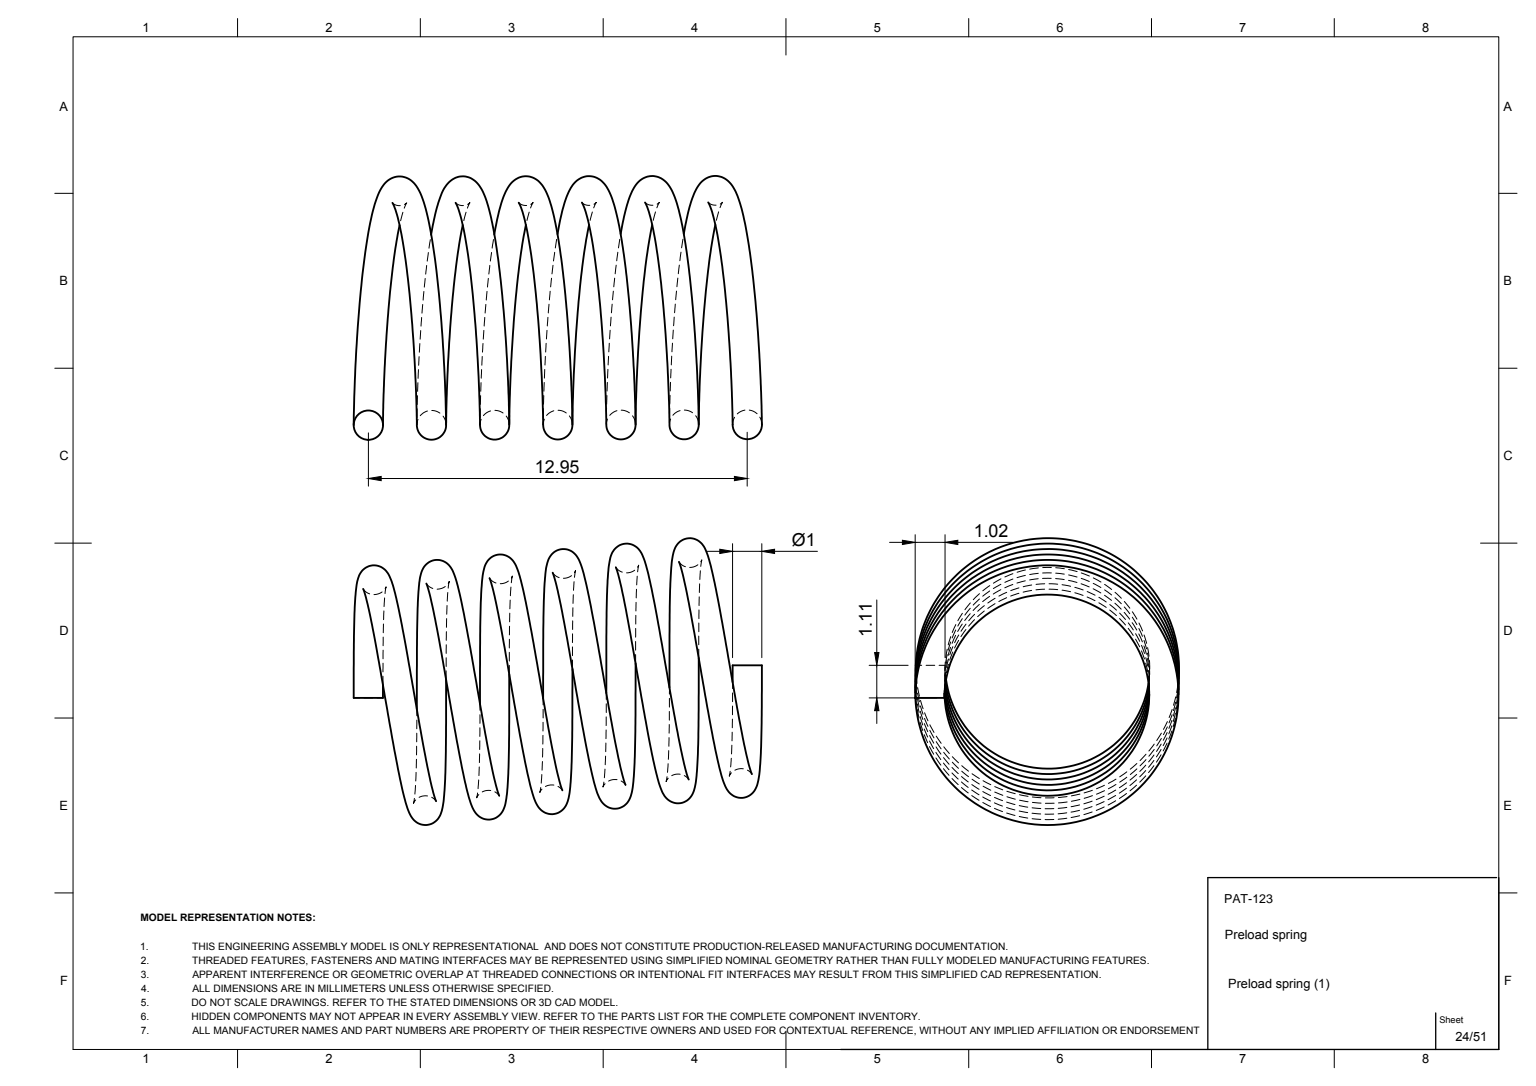
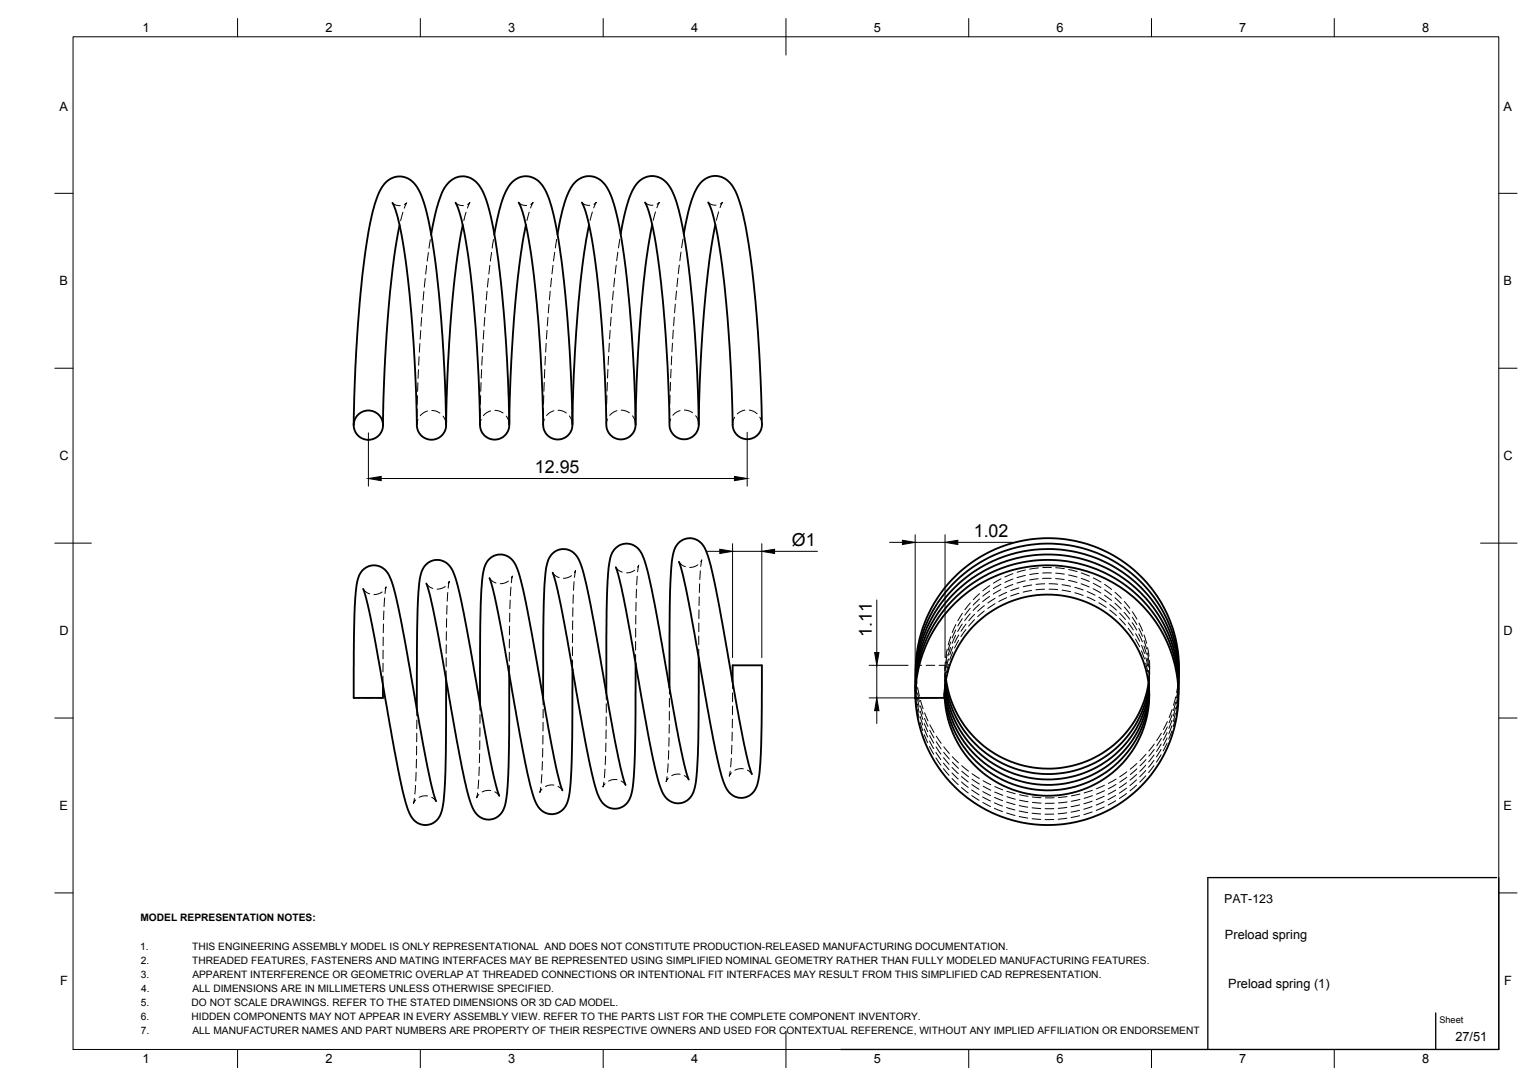
ISO-10303-21;
HEADER;
/* Generated by software containing ST-Developer
 * from STEP Tools, Inc. (www.steptools.com) 
 */

FILE_DESCRIPTION(
/* description */ ('Worm-less right-angle friction wheel drive'),
/* implementation_level */ '2;1');

FILE_NAME(
/* name */ 'Preload spring (1).step',
/* time_stamp */ '2026-10-28T03:22:36-07:00',
/* author */ (''),
/* organization */ (''),
/* preprocessor_version */ 'ST-DEVELOPER v20.2',
/* originating_system */ 'Autodesk Translation Framework v15.17.0.0',
/* authorisation */ '');

FILE_SCHEMA (('AUTOMOTIVE_DESIGN { 1 0 10303 214 3 1 1 }'));
ENDSEC;

DATA;
#10=MECHANICAL_DESIGN_GEOMETRIC_PRESENTATION_REPRESENTATION('',(#633),#17046);
#482=B_SPLINE_CURVE_WITH_KNOTS('',3,(#15240,#15241,#15242,#15243,#15244,
#15245,#15246,#15247,#15248,#15249,#15250,#15251,#15252,#15253,#15254,#15255,
#15256,#15257,#15258,#15259,#15260,#15261,#15262,#15263,#15264,#15265,#15266,
#15267,#15268,#15269,#15270,#15271,#15272,#15273,#15274,#15275,#15276,#15277,
#15278,#15279,#15280,#15281,#15282,#15283,#15284,#15285,#15286,#15287,#15288,
#15289,#15290,#15291,#15292,#15293,#15294,#15295,#15296,#15297,#15298,#15299,
#15300,#15301,#15302,#15303,#15304,#15305,#15306,#15307,#15308,#15309,#15310,
#15311,#15312,#15313,#15314,#15315,#15316,#15317,#15318,#15319,#15320),
 .UNSPECIFIED.,.F.,.F.,(4,1,1,1,1,1,1,1,1,1,1,1,1,1,1,1,1,1,1,1,1,1,1,1,
1,1,1,1,1,1,1,1,1,1,1,1,1,1,1,1,1,1,1,1,1,1,1,1,1,1,1,1,1,1,1,1,1,1,1,1,
1,1,1,1,1,1,1,1,1,1,1,1,1,1,1,1,1,1,4),(0.,0.00892857142857143,0.0178571428571429,
0.0357142857142857,0.0535714285714286,0.0714285714285714,0.0892857142857143,
0.107142857142857,0.125,0.142857142857143,0.158730158730159,0.174603174603175,
0.19047619047619,0.202380952380952,0.214285714285714,0.220238095238095,
0.226190476190476,0.238095238095238,0.25,0.261904761904762,0.273809523809524,
0.285714285714286,0.297619047619048,0.30952380952381,0.321428571428571,
0.333333333333333,0.349206349206349,0.365079365079365,0.376984126984127,
0.380952380952381,0.392857142857143,0.404761904761905,0.416666666666667,
0.428571428571429,0.446428571428571,0.464285714285714,0.476190476190476,
0.485119047619048,0.5,0.508928571428571,0.517857142857143,0.535714285714286,
0.553571428571429,0.571428571428571,0.589285714285714,0.607142857142857,
0.625,0.642857142857143,0.651785714285714,0.654761904761905,0.666666666666667,
0.678571428571428,0.696428571428571,0.705357142857143,0.714285714285714,
0.726190476190476,0.738095238095238,0.75,0.761904761904762,0.773809523809524,
0.785714285714286,0.797619047619047,0.803571428571428,0.806547619047619,
0.809523809523809,0.821428571428571,0.833333333333333,0.845238095238095,
0.857142857142857,0.866071428571429,0.875,0.892857142857143,0.910714285714286,
0.928571428571429,0.946428571428571,0.964285714285714,0.982142857142857,
0.991071428571429,1.),.UNSPECIFIED.);
#516=B_SPLINE_SURFACE_WITH_KNOTS('',3,3,((#14427,#14428,#14429,#14430,#14431,
#14432,#14433,#14434,#14435,#14436,#14437,#14438,#14439,#14440,#14441,#14442,
#14443,#14444,#14445,#14446,#14447,#14448,#14449,#14450,#14451,#14452,#14453,
#14454,#14455,#14456,#14457,#14458,#14459,#14460,#14461,#14462,#14463,#14464,
#14465,#14466,#14467,#14468,#14469,#14470,#14471,#14472,#14473,#14474,#14475,
#14476,#14477,#14478,#14479,#14480,#14481,#14482,#14483,#14484,#14485,#14486,
#14487,#14488,#14489,#14490,#14491,#14492,#14493,#14494,#14495,#14496,#14497,
#14498,#14499,#14500,#14501,#14502,#14503,#14504,#14505,#14506,#14507),
(#14508,#14509,#14510,#14511,#14512,#14513,#14514,#14515,#14516,#14517,
#14518,#14519,#14520,#14521,#14522,#14523,#14524,#14525,#14526,#14527,#14528,
#14529,#14530,#14531,#14532,#14533,#14534,#14535,#14536,#14537,#14538,#14539,
#14540,#14541,#14542,#14543,#14544,#14545,#14546,#14547,#14548,#14549,#14550,
#14551,#14552,#14553,#14554,#14555,#14556,#14557,#14558,#14559,#14560,#14561,
#14562,#14563,#14564,#14565,#14566,#14567,#14568,#14569,#14570,#14571,#14572,
#14573,#14574,#14575,#14576,#14577,#14578,#14579,#14580,#14581,#14582,#14583,
#14584,#14585,#14586,#14587,#14588),(#14589,#14590,#14591,#14592,#14593,
#14594,#14595,#14596,#14597,#14598,#14599,#14600,#14601,#14602,#14603,#14604,
#14605,#14606,#14607,#14608,#14609,#14610,#14611,#14612,#14613,#14614,#14615,
#14616,#14617,#14618,#14619,#14620,#14621,#14622,#14623,#14624,#14625,#14626,
#14627,#14628,#14629,#14630,#14631,#14632,#14633,#14634,#14635,#14636,#14637,
#14638,#14639,#14640,#14641,#14642,#14643,#14644,#14645,#14646,#14647,#14648,
#14649,#14650,#14651,#14652,#14653,#14654,#14655,#14656,#14657,#14658,#14659,
#14660,#14661,#14662,#14663,#14664,#14665,#14666,#14667,#14668,#14669),
(#14670,#14671,#14672,#14673,#14674,#14675,#14676,#14677,#14678,#14679,
#14680,#14681,#14682,#14683,#14684,#14685,#14686,#14687,#14688,#14689,#14690,
#14691,#14692,#14693,#14694,#14695,#14696,#14697,#14698,#14699,#14700,#14701,
#14702,#14703,#14704,#14705,#14706,#14707,#14708,#14709,#14710,#14711,#14712,
#14713,#14714,#14715,#14716,#14717,#14718,#14719,#14720,#14721,#14722,#14723,
#14724,#14725,#14726,#14727,#14728,#14729,#14730,#14731,#14732,#14733,#14734,
#14735,#14736,#14737,#14738,#14739,#14740,#14741,#14742,#14743,#14744,#14745,
#14746,#14747,#14748,#14749,#14750),(#14751,#14752,#14753,#14754,#14755,
#14756,#14757,#14758,#14759,#14760,#14761,#14762,#14763,#14764,#14765,#14766,
#14767,#14768,#14769,#14770,#14771,#14772,#14773,#14774,#14775,#14776,#14777,
#14778,#14779,#14780,#14781,#14782,#14783,#14784,#14785,#14786,#14787,#14788,
#14789,#14790,#14791,#14792,#14793,#14794,#14795,#14796,#14797,#14798,#14799,
#14800,#14801,#14802,#14803,#14804,#14805,#14806,#14807,#14808,#14809,#14810,
#14811,#14812,#14813,#14814,#14815,#14816,#14817,#14818,#14819,#14820,#14821,
#14822,#14823,#14824,#14825,#14826,#14827,#14828,#14829,#14830,#14831),
(#14832,#14833,#14834,#14835,#14836,#14837,#14838,#14839,#14840,#14841,
#14842,#14843,#14844,#14845,#14846,#14847,#14848,#14849,#14850,#14851,#14852,
#14853,#14854,#14855,#14856,#14857,#14858,#14859,#14860,#14861,#14862,#14863,
#14864,#14865,#14866,#14867,#14868,#14869,#14870,#14871,#14872,#14873,#14874,
#14875,#14876,#14877,#14878,#14879,#14880,#14881,#14882,#14883,#14884,#14885,
#14886,#14887,#14888,#14889,#14890,#14891,#14892,#14893,#14894,#14895,#14896,
#14897,#14898,#14899,#14900,#14901,#14902,#14903,#14904,#14905,#14906,#14907,
#14908,#14909,#14910,#14911,#14912),(#14913,#14914,#14915,#14916,#14917,
#14918,#14919,#14920,#14921,#14922,#14923,#14924,#14925,#14926,#14927,#14928,
#14929,#14930,#14931,#14932,#14933,#14934,#14935,#14936,#14937,#14938,#14939,
#14940,#14941,#14942,#14943,#14944,#14945,#14946,#14947,#14948,#14949,#14950,
#14951,#14952,#14953,#14954,#14955,#14956,#14957,#14958,#14959,#14960,#14961,
#14962,#14963,#14964,#14965,#14966,#14967,#14968,#14969,#14970,#14971,#14972,
#14973,#14974,#14975,#14976,#14977,#14978,#14979,#14980,#14981,#14982,#14983,
#14984,#14985,#14986,#14987,#14988,#14989,#14990,#14991,#14992,#14993),
(#14994,#14995,#14996,#14997,#14998,#14999,#15000,#15001,#15002,#15003,
#15004,#15005,#15006,#15007,#15008,#15009,#15010,#15011,#15012,#15013,#15014,
#15015,#15016,#15017,#15018,#15019,#15020,#15021,#15022,#15023,#15024,#15025,
#15026,#15027,#15028,#15029,#15030,#15031,#15032,#15033,#15034,#15035,#15036,
#15037,#15038,#15039,#15040,#15041,#15042,#15043,#15044,#15045,#15046,#15047,
#15048,#15049,#15050,#15051,#15052,#15053,#15054,#15055,#15056,#15057,#15058,
#15059,#15060,#15061,#15062,#15063,#15064,#15065,#15066,#15067,#15068,#15069,
#15070,#15071,#15072,#15073,#15074),(#15075,#15076,#15077,#15078,#15079,
#15080,#15081,#15082,#15083,#15084,#15085,#15086,#15087,#15088,#15089,#15090,
#15091,#15092,#15093,#15094,#15095,#15096,#15097,#15098,#15099,#15100,#15101,
#15102,#15103,#15104,#15105,#15106,#15107,#15108,#15109,#15110,#15111,#15112,
#15113,#15114,#15115,#15116,#15117,#15118,#15119,#15120,#15121,#15122,#15123,
#15124,#15125,#15126,#15127,#15128,#15129,#15130,#15131,#15132,#15133,#15134,
#15135,#15136,#15137,#15138,#15139,#15140,#15141,#15142,#15143,#15144,#15145,
#15146,#15147,#15148,#15149,#15150,#15151,#15152,#15153,#15154,#15155),
(#15156,#15157,#15158,#15159,#15160,#15161,#15162,#15163,#15164,#15165,
#15166,#15167,#15168,#15169,#15170,#15171,#15172,#15173,#15174,#15175,#15176,
#15177,#15178,#15179,#15180,#15181,#15182,#15183,#15184,#15185,#15186,#15187,
#15188,#15189,#15190,#15191,#15192,#15193,#15194,#15195,#15196,#15197,#15198,
#15199,#15200,#15201,#15202,#15203,#15204,#15205,#15206,#15207,#15208,#15209,
#15210,#15211,#15212,#15213,#15214,#15215,#15216,#15217,#15218,#15219,#15220,
#15221,#15222,#15223,#15224,#15225,#15226,#15227,#15228,#15229,#15230,#15231,
#15232,#15233,#15234,#15235,#15236)),.UNSPECIFIED.,.T.,.F.,.F.,(4,1,1,1,
1,1,1,4),(4,1,1,1,1,1,1,1,1,1,1,1,1,1,1,1,1,1,1,1,1,1,1,1,1,1,1,1,1,1,1,
1,1,1,1,1,1,1,1,1,1,1,1,1,1,1,1,1,1,1,1,1,1,1,1,1,1,1,1,1,1,1,1,1,1,1,1,
1,1,1,1,1,1,1,1,1,1,1,4),(-3.14159265358979,-2.24399475256414,-1.34639685153848,
-0.448798950512828,0.448798950512828,1.34639685153848,2.24399475256414,
3.14159265358979),(0.,0.00892857142857143,0.0178571428571429,0.0357142857142857,
0.0535714285714286,0.0714285714285714,0.0892857142857143,0.107142857142857,
0.125,0.142857142857143,0.158730158730159,0.174603174603175,0.19047619047619,
0.202380952380952,0.214285714285714,0.220238095238095,0.226190476190476,
0.238095238095238,0.25,0.261904761904762,0.273809523809524,0.285714285714286,
0.297619047619048,0.30952380952381,0.321428571428571,0.333333333333333,
0.349206349206349,0.365079365079365,0.376984126984127,0.380952380952381,
0.392857142857143,0.404761904761905,0.416666666666667,0.428571428571429,
0.446428571428571,0.464285714285714,0.476190476190476,0.485119047619048,
0.5,0.508928571428571,0.517857142857143,0.535714285714286,0.553571428571429,
0.571428571428571,0.589285714285714,0.607142857142857,0.625,0.642857142857143,
0.651785714285714,0.654761904761905,0.666666666666667,0.678571428571428,
0.696428571428571,0.705357142857143,0.714285714285714,0.726190476190476,
0.738095238095238,0.75,0.761904761904762,0.773809523809524,0.785714285714286,
0.797619047619047,0.803571428571428,0.806547619047619,0.809523809523809,
0.821428571428571,0.833333333333333,0.845238095238095,0.857142857142857,
0.866071428571429,0.875,0.892857142857143,0.910714285714286,0.928571428571429,
0.946428571428571,0.964285714285714,0.982142857142857,0.991071428571429,
1.),.UNSPECIFIED.);
#539=SHAPE_REPRESENTATION_RELATIONSHIP('SRR','None',#17282,#586);
#586=ADVANCED_BREP_SHAPE_REPRESENTATION('',(#687),#17018);
#633=STYLED_ITEM('',(#17591),#687);
#687=MANIFOLD_SOLID_BREP('Body1',#8188);
#1066=PLANE('',#9233);
#1067=PLANE('',#9234);
#1439=FACE_OUTER_BOUND('',#2095,.T.);
#1440=FACE_OUTER_BOUND('',#2096,.T.);
#1441=FACE_OUTER_BOUND('',#2097,.T.);
#2095=EDGE_LOOP('',(#6596,#6597,#6598,#6599));
#2096=EDGE_LOOP('',(#6600));
#2097=EDGE_LOOP('',(#6601));
#3691=CIRCLE('',#9231,0.05);
#3692=CIRCLE('',#9232,0.05);
#4223=VERTEX_POINT('',#15237);
#4224=VERTEX_POINT('',#15239);
#5067=EDGE_CURVE('',#4223,#4223,#3691,.T.);
#5068=EDGE_CURVE('',#4223,#4224,#482,.T.);
#5069=EDGE_CURVE('',#4224,#4224,#3692,.T.);
#6596=ORIENTED_EDGE('',*,*,#5067,.T.);
#6597=ORIENTED_EDGE('',*,*,#5068,.T.);
#6598=ORIENTED_EDGE('',*,*,#5069,.F.);
#6599=ORIENTED_EDGE('',*,*,#5068,.F.);
#6600=ORIENTED_EDGE('',*,*,#5069,.T.);
#6601=ORIENTED_EDGE('',*,*,#5067,.F.);
#7931=ADVANCED_FACE('',(#1439),#516,.T.);
#7932=ADVANCED_FACE('',(#1440),#1066,.T.);
#7933=ADVANCED_FACE('',(#1441),#1067,.F.);
#8188=CLOSED_SHELL('',(#7931,#7932,#7933));
#9230=AXIS2_PLACEMENT_3D('',#14426,#11045,#11046);
#9231=AXIS2_PLACEMENT_3D('',#15238,#11047,#11048);
#9232=AXIS2_PLACEMENT_3D('',#15321,#11049,#11050);
#9233=AXIS2_PLACEMENT_3D('',#15322,#11051,#11052);
#9234=AXIS2_PLACEMENT_3D('',#15323,#11053,#11054);
#11045=DIRECTION('axis',(0.,0.,1.));
#11046=DIRECTION('refdir',(1.,0.,0.));
#11047=DIRECTION('center_axis',(-0.000134420183300025,-0.085636011539688,
0.996326480356107));
#11048=DIRECTION('ref_axis',(1.1553650826854E-5,-0.996326489423811,-0.0856360107603029));
#11049=DIRECTION('center_axis',(0.000134419999317792,-0.085636011399563,
0.996326480368176));
#11050=DIRECTION('ref_axis',(0.0962365814952688,0.991703136101715,0.0852256430197378));
#11051=DIRECTION('center_axis',(0.000134419999317792,-0.085636011399563,
0.996326480368176));
#11052=DIRECTION('ref_axis',(0.0962365814952688,0.991703136101715,0.0852256430197378));
#11053=DIRECTION('center_axis',(-0.000134420183300025,-0.085636011539688,
0.996326480356107));
#11054=DIRECTION('ref_axis',(1.1553650826854E-5,-0.996326489423811,-0.0856360107603029));
#14426=CARTESIAN_POINT('',(0.,0.,0.));
#14427=CARTESIAN_POINT('Ctrl Pts',(5.89999942231746,7.09981632447119,4.00428180053801));
#14428=CARTESIAN_POINT('Ctrl Pts',(5.89999334367971,7.09594376396835,4.04933684813297));
#14429=CARTESIAN_POINT('Ctrl Pts',(5.88465017335476,7.08819405075721,4.13908165517953));
#14430=CARTESIAN_POINT('Ctrl Pts',(5.7964860030169,7.07263331806119,4.29968204261715));
#14431=CARTESIAN_POINT('Ctrl Pts',(5.59351456200701,7.05308119240215,4.4275031391656));
#14432=CARTESIAN_POINT('Ctrl Pts',(5.30510775645105,7.02945158726801,4.39546636939848));
#14433=CARTESIAN_POINT('Ctrl Pts',(5.09844717527872,7.00565845259414,4.18908156433879));
#14434=CARTESIAN_POINT('Ctrl Pts',(5.06491507736497,6.98170283632427,3.89688445847127));
#14435=CARTESIAN_POINT('Ctrl Pts',(5.22229231109316,6.957587725778,3.64598811283775));
#14436=CARTESIAN_POINT('Ctrl Pts',(5.50350105188817,6.93331581944121,3.54720017800962));
#14437=CARTESIAN_POINT('Ctrl Pts',(5.77606730494162,6.90979543600253,3.64243302852389));
#14438=CARTESIAN_POINT('Ctrl Pts',(5.93155863446605,6.88704927881041,3.87048202703801));
#14439=CARTESIAN_POINT('Ctrl Pts',(5.93201459027321,6.86509833940111,4.13672884061229));
#14440=CARTESIAN_POINT('Ctrl Pts',(5.79395734371705,6.84487476341531,4.33956419787309));
#14441=CARTESIAN_POINT('Ctrl Pts',(5.59585169142646,6.82641140225049,4.43472796239094));
#14442=CARTESIAN_POINT('Ctrl Pts',(5.43062330290708,6.81251496798271,4.43483227755276));
#14443=CARTESIAN_POINT('Ctrl Pts',(5.30781628774365,6.8013693608627,4.39175312056372));
#14444=CARTESIAN_POINT('Ctrl Pts',(5.19743069189207,6.79020509173472,4.32251414855249));
#14445=CARTESIAN_POINT('Ctrl Pts',(5.09353798605695,6.77621535562195,4.1924772803632));
#14446=CARTESIAN_POINT('Ctrl Pts',(5.04898925851302,6.75937456735607,3.99715324700454));
#14447=CARTESIAN_POINT('Ctrl Pts',(5.0935413464267,6.74248271039737,3.80123524176677));
#14448=CARTESIAN_POINT('Ctrl Pts',(5.21917592334569,6.72554188446977,3.64363320271165));
#14449=CARTESIAN_POINT('Ctrl Pts',(5.40122000385758,6.70855426693318,3.55590244763416));
#14450=CARTESIAN_POINT('Ctrl Pts',(5.60380955719718,6.6915221019177,3.55584448787041));
#14451=CARTESIAN_POINT('Ctrl Pts',(5.78691645390742,6.67444770371231,3.64394104146688));
#14452=CARTESIAN_POINT('Ctrl Pts',(5.91372041331327,6.65733344366189,3.80307026683985));
#14453=CARTESIAN_POINT('Ctrl Pts',(5.96466327221314,6.63827601600008,4.02414934139344));
#14454=CARTESIAN_POINT('Ctrl Pts',(5.88961383686182,6.61726302422527,4.26770951451258));
#14455=CARTESIAN_POINT('Ctrl Pts',(5.68975602864846,6.59619863118807,4.42707389952551));
#14456=CARTESIAN_POINT('Ctrl Pts',(5.50916223586277,6.58084997697241,4.45396467698472));
#14457=CARTESIAN_POINT('Ctrl Pts',(5.35453310810722,6.56740673736238,4.43070717074375));
#14458=CARTESIAN_POINT('Ctrl Pts',(5.21033393748589,6.55395079494006,4.36132595428699));
#14459=CARTESIAN_POINT('Ctrl Pts',(5.08177516019845,6.53662851034176,4.20021226638331));
#14460=CARTESIAN_POINT('Ctrl Pts',(5.03609211123456,6.51928717867399,3.99913913108666));
#14461=CARTESIAN_POINT('Ctrl Pts',(5.08928582945947,6.49903664031616,3.76419897777231));
#14462=CARTESIAN_POINT('Ctrl Pts',(5.28978283301087,6.47587070029814,3.56256415950519));
#14463=CARTESIAN_POINT('Ctrl Pts',(5.57279015344961,6.4526862562021,3.53101713469425));
#14464=CARTESIAN_POINT('Ctrl Pts',(5.7744501239661,6.4338421384389,3.62890875798563));
#14465=CARTESIAN_POINT('Ctrl Pts',(5.91107614262552,6.41644569471267,3.78134048060785));
#14466=CARTESIAN_POINT('Ctrl Pts',(5.96451577569518,6.40049895608791,3.96616344909838));
#14467=CARTESIAN_POINT('Ctrl Pts',(5.9327299609379,6.3845554854669,4.15104965949736));
#14468=CARTESIAN_POINT('Ctrl Pts',(5.83415684595966,6.36716688464879,4.33040203531341));
#14469=CARTESIAN_POINT('Ctrl Pts',(5.60855787080152,6.3454421500065,4.47243154476512));
#14470=CARTESIAN_POINT('Ctrl Pts',(5.29067075546292,6.31939963984916,4.43654609473001));
#14471=CARTESIAN_POINT('Ctrl Pts',(5.06495666340114,6.29339375333233,4.21070709279472));
#14472=CARTESIAN_POINT('Ctrl Pts',(5.02940089438198,6.26743382198568,3.89407398616837));
#14473=CARTESIAN_POINT('Ctrl Pts',(5.19880065125732,6.24152902171826,3.62471661866899));
#14474=CARTESIAN_POINT('Ctrl Pts',(5.49820781434257,6.21568834443117,3.52014376389726));
#14475=CARTESIAN_POINT('Ctrl Pts',(5.74701061020189,6.19421520170402,3.60728770872527));
#14476=CARTESIAN_POINT('Ctrl Pts',(5.85863359577984,6.17993370216935,3.73296424281348));
#14477=CARTESIAN_POINT('Ctrl Pts',(5.92288006435656,6.16852118154694,3.84896516413552));
#14478=CARTESIAN_POINT('Ctrl Pts',(5.95664235896203,6.15570021350747,3.99755228818456));
#14479=CARTESIAN_POINT('Ctrl Pts',(5.90422907170185,6.13580438066566,4.22863954557107));
#14480=CARTESIAN_POINT('Ctrl Pts',(5.74463079333177,6.1173884553624,4.38823789360272));
#14481=CARTESIAN_POINT('Ctrl Pts',(5.55259803695828,6.10044178794059,4.44287010078724));
#14482=CARTESIAN_POINT('Ctrl Pts',(5.38717753744307,6.08634982964905,4.43381260797737));
#14483=CARTESIAN_POINT('Ctrl Pts',(5.22149962135128,6.07088880373497,4.35387124517548));
#14484=CARTESIAN_POINT('Ctrl Pts',(5.09676922730111,6.0540743240685,4.197519449458));
#14485=CARTESIAN_POINT('Ctrl Pts',(5.0525318165955,6.03731392845979,4.00312051246728));
#14486=CARTESIAN_POINT('Ctrl Pts',(5.09677460214568,6.02060952469266,3.80936725739853));
#14487=CARTESIAN_POINT('Ctrl Pts',(5.22036100773764,6.00396293698029,3.65469518694587));
#14488=CARTESIAN_POINT('Ctrl Pts',(5.39815221757406,5.98737590584214,3.56901265908242));
#14489=CARTESIAN_POINT('Ctrl Pts',(5.56194673621828,5.9736043825902,3.56918712785721));
#14490=CARTESIAN_POINT('Ctrl Pts',(5.6678409475086,5.96399177625527,3.60634259138081));
#14491=CARTESIAN_POINT('Ctrl Pts',(5.72360710674561,5.9585067948969,3.63716464071472));
#14492=CARTESIAN_POINT('Ctrl Pts',(5.80152037634414,5.9502873075744,3.69239994875946));
#14493=CARTESIAN_POINT('Ctrl Pts',(5.89262775771971,5.93798818799799,3.80682412790902));
#14494=CARTESIAN_POINT('Ctrl Pts',(5.93588165070209,5.9216549676263,3.9962737943898));
#14495=CARTESIAN_POINT('Ctrl Pts',(5.89265315890838,5.90538862230925,4.18485446150754));
#14496=CARTESIAN_POINT('Ctrl Pts',(5.78249899819111,5.89054018760752,4.32296861862104));
#14497=CARTESIAN_POINT('Ctrl Pts',(5.64397324912796,5.87709200642215,4.39928196165792));
#14498=CARTESIAN_POINT('Ctrl Pts',(5.45729571883929,5.86100659113963,4.43140768516966));
#14499=CARTESIAN_POINT('Ctrl Pts',(5.22574876053333,5.84099901355926,4.35024097908663));
#14500=CARTESIAN_POINT('Ctrl Pts',(5.0699063365284,5.81715142001874,4.10208650989737));
#14501=CARTESIAN_POINT('Ctrl Pts',(5.10298913581097,5.79346725679344,3.81314318112568));
#14502=CARTESIAN_POINT('Ctrl Pts',(5.30729513304354,5.76994860790156,3.60917536341897));
#14503=CARTESIAN_POINT('Ctrl Pts',(5.59246492988907,5.74659517888843,3.57738640664907));
#14504=CARTESIAN_POINT('Ctrl Pts',(5.79284572265032,5.72727468967069,3.7038989587173));
#14505=CARTESIAN_POINT('Ctrl Pts',(5.8800308145667,5.71189869700794,3.86253471396896));
#14506=CARTESIAN_POINT('Ctrl Pts',(5.8951821641861,5.70424160396714,3.95121652410008));
#14507=CARTESIAN_POINT('Ctrl Pts',(5.89518817092524,5.70041484319491,3.99573871784903));
#14508=CARTESIAN_POINT('Ctrl Pts',(5.88503945743652,7.09981632447119,4.0042797822024));
#14509=CARTESIAN_POINT('Ctrl Pts',(5.88503360188162,7.09608588493208,4.04768133289771));
#14510=CARTESIAN_POINT('Ctrl Pts',(5.87026126699026,7.08862396394419,4.13409876124989));
#14511=CARTESIAN_POINT('Ctrl Pts',(5.78535030584819,7.07363703375696,4.28878882173021));
#14512=CARTESIAN_POINT('Ctrl Pts',(5.58981457160439,7.05480252942765,4.41195005833011));
#14513=CARTESIAN_POINT('Ctrl Pts',(5.31179486198712,7.03202561227573,4.38109726858311));
#14514=CARTESIAN_POINT('Ctrl Pts',(5.1124277587765,7.00907674704486,4.18203908678982));
#14515=CARTESIAN_POINT('Ctrl Pts',(5.08001803350251,6.98595417860409,3.8999761925135));
#14516=CARTESIAN_POINT('Ctrl Pts',(5.23203136694347,6.96266049576345,3.65754564919961));
#14517=CARTESIAN_POINT('Ctrl Pts',(5.50396936937568,6.93919148734548,3.56195831409131));
#14518=CARTESIAN_POINT('Ctrl Pts',(5.76786360761367,6.91642620730754,3.65410210166395));
#14519=CARTESIAN_POINT('Ctrl Pts',(5.91859875131219,6.89438580758112,3.87509306663505));
#14520=CARTESIAN_POINT('Ctrl Pts',(5.91908754056048,6.8730906966479,4.13341261767347));
#14521=CARTESIAN_POINT('Ctrl Pts',(5.78502683264549,6.85345041326714,4.33045812820945));
#14522=CARTESIAN_POINT('Ctrl Pts',(5.59240862903414,6.83550085128541,4.42301346486046));
#14523=CARTESIAN_POINT('Ctrl Pts',(5.43159993473068,6.82197903313836,4.42313220394627));
#14524=CARTESIAN_POINT('Ctrl Pts',(5.31198346558657,6.81112423395334,4.38117622245278));
#14525=CARTESIAN_POINT('Ctrl Pts',(5.20441120090185,6.80024507289894,4.31370604089673));
#14526=CARTESIAN_POINT('Ctrl Pts',(5.10308448889811,6.78660773456135,4.18691472624338));
#14527=CARTESIAN_POINT('Ctrl Pts',(5.05957333477074,6.7701692409416,3.99624133185818));
#14528=CARTESIAN_POINT('Ctrl Pts',(5.10308658178506,6.75366451037247,3.80477816416283));
#14529=CARTESIAN_POINT('Ctrl Pts',(5.22596911064028,6.73709691740872,3.65058727641187));
#14530=CARTESIAN_POINT('Ctrl Pts',(5.40424154502889,6.72046420161793,3.56464409931812));
#14531=CARTESIAN_POINT('Ctrl Pts',(5.60286757635272,6.70376966024345,3.56456110898369));
#14532=CARTESIAN_POINT('Ctrl Pts',(5.78260975317895,6.68701499206993,3.65100600925544));
#14533=CARTESIAN_POINT('Ctrl Pts',(5.90723898021823,6.67020103323329,3.80736557672115));
#14534=CARTESIAN_POINT('Ctrl Pts',(5.95739144160597,6.65145878281361,4.02485643420641));
#14535=CARTESIAN_POINT('Ctrl Pts',(5.88350382080552,6.63075660525971,4.26484435626206));
#14536=CARTESIAN_POINT('Ctrl Pts',(5.68632699032047,6.60997572305765,4.42215495861284));
#14537=CARTESIAN_POINT('Ctrl Pts',(5.50786242867171,6.59481082042869,4.44875398416139));
#14538=CARTESIAN_POINT('Ctrl Pts',(5.35492443239398,6.58151601836513,4.42575382239937));
#14539=CARTESIAN_POINT('Ctrl Pts',(5.21218195064913,6.56819993097658,4.35709671903736));
#14540=CARTESIAN_POINT('Ctrl Pts',(5.08473882673911,6.55103208305566,4.19743115221831));
#14541=CARTESIAN_POINT('Ctrl Pts',(5.03937938103974,6.53382903633989,3.9979075972426));
#14542=CARTESIAN_POINT('Ctrl Pts',(5.09219616215328,6.51371045047149,3.76446604094244));
#14543=CARTESIAN_POINT('Ctrl Pts',(5.29164216583296,6.49066863108082,3.56375987550904));
#14544=CARTESIAN_POINT('Ctrl Pts',(5.57380855674231,6.46755668746403,3.53221661138612));
#14545=CARTESIAN_POINT('Ctrl Pts',(5.77520948735709,6.44874487708301,3.62994883143992));
#14546=CARTESIAN_POINT('Ctrl Pts',(5.9118194085888,6.4313515231649,3.78234207954662));
#14547=CARTESIAN_POINT('Ctrl Pts',(5.96535290798642,6.41539494756269,3.96733324055338));
#14548=CARTESIAN_POINT('Ctrl Pts',(5.93350724448179,6.39941600080786,4.15265573762338));
#14549=CARTESIAN_POINT('Ctrl Pts',(5.83462795102543,6.38197230496921,4.3326009207179));
#14550=CARTESIAN_POINT('Ctrl Pts',(5.60802480207367,6.36015239803693,4.47536066940383));
#14551=CARTESIAN_POINT('Ctrl Pts',(5.28804071704905,6.33394375008401,4.43934003157992));
#14552=CARTESIAN_POINT('Ctrl Pts',(5.0603505371736,6.30772509227727,4.2116637907064));
#14553=CARTESIAN_POINT('Ctrl Pts',(5.02433426469034,6.28150024364713,3.89177497027619));
#14554=CARTESIAN_POINT('Ctrl Pts',(5.19569399285247,6.25529612930055,3.61911293303289));
#14555=CARTESIAN_POINT('Ctrl Pts',(5.49925070212339,6.22909620166617,3.51299220778051));
#14556=CARTESIAN_POINT('Ctrl Pts',(5.75197475889608,6.20729451095337,3.60142940412264));
#14557=CARTESIAN_POINT('Ctrl Pts',(5.86550798533523,6.19277158813603,3.72923955502794));
#14558=CARTESIAN_POINT('Ctrl Pts',(5.93088617148282,6.18115900724412,3.8472804234726));
#14559=CARTESIAN_POINT('Ctrl Pts',(5.96528306606778,6.16810503068496,3.99858218016166));
#14560=CARTESIAN_POINT('Ctrl Pts',(5.91188622152517,6.14782425772989,4.23416182125941));
#14561=CARTESIAN_POINT('Ctrl Pts',(5.7490193624655,6.12903078679408,4.39711001697646));
#14562=CARTESIAN_POINT('Ctrl Pts',(5.55277074738954,6.11171437387845,4.45295636322444));
#14563=CARTESIAN_POINT('Ctrl Pts',(5.38358725567555,6.09730363521905,4.44370269520848));
#14564=CARTESIAN_POINT('Ctrl Pts',(5.21398497489651,6.08147921618268,4.3618860003188));
#14565=CARTESIAN_POINT('Ctrl Pts',(5.08616324600684,6.06425310299918,4.20169628716414));
#14566=CARTESIAN_POINT('Ctrl Pts',(5.04077402087937,6.04706393365499,4.00231532025332));
#14567=CARTESIAN_POINT('Ctrl Pts',(5.08617032093218,6.02991837734054,3.80341237994541));
#14568=CARTESIAN_POINT('Ctrl Pts',(5.21314140461402,6.01281654577742,3.64447952839659));
#14569=CARTESIAN_POINT('Ctrl Pts',(5.39596558147649,5.99576114159946,3.55635140588749));
#14570=CARTESIAN_POINT('Ctrl Pts',(5.56454843416681,5.98158811350942,3.55651828149823));
#14571=CARTESIAN_POINT('Ctrl Pts',(5.67360413989068,5.97168893571421,3.59478043709277));
#14572=CARTESIAN_POINT('Ctrl Pts',(5.73105166386915,5.96603869488852,3.62653169595776));
#14573=CARTESIAN_POINT('Ctrl Pts',(5.8113292722746,5.95756999758158,3.68344222347348));
#14574=CARTESIAN_POINT('Ctrl Pts',(5.90525200105339,5.94489303633764,3.80138469729133));
#14575=CARTESIAN_POINT('Ctrl Pts',(5.9498859624265,5.92804546902486,3.99680740667185));
#14576=CARTESIAN_POINT('Ctrl Pts',(5.90527406073601,5.91125567170158,4.19147367065731));
#14577=CARTESIAN_POINT('Ctrl Pts',(5.79150254559316,5.89591895994826,4.33414205895609));
#14578=CARTESIAN_POINT('Ctrl Pts',(5.64834101429215,5.88202102372911,4.4130140624278));
#14579=CARTESIAN_POINT('Ctrl Pts',(5.4553346472487,5.86539043683629,4.44623569719961));
#14580=CARTESIAN_POINT('Ctrl Pts',(5.21578000821573,5.84469228785158,4.36229253299229));
#14581=CARTESIAN_POINT('Ctrl Pts',(5.05441367332187,5.82000362720346,4.10540136247045));
#14582=CARTESIAN_POINT('Ctrl Pts',(5.08866429485251,5.79546931039049,3.80607791306765));
#14583=CARTESIAN_POINT('Ctrl Pts',(5.30040509492993,5.77109351117434,3.59466769610795));
#14584=CARTESIAN_POINT('Ctrl Pts',(5.59608563803559,5.74687955036343,3.56169371934204));
#14585=CARTESIAN_POINT('Ctrl Pts',(5.80392030130352,5.72684060107471,3.69290766840958));
#14586=CARTESIAN_POINT('Ctrl Pts',(5.89435424813677,5.71089217884313,3.85744883447212));
#14587=CARTESIAN_POINT('Ctrl Pts',(5.91007247017572,5.70294882509164,3.94944546934017));
#14588=CARTESIAN_POINT('Ctrl Pts',(5.91007869895502,5.69898060743533,3.99561343380099));
#14589=CARTESIAN_POINT('Ctrl Pts',(5.85520827475736,7.08553591511819,4.00304833122987));
#14590=CARTESIAN_POINT('Ctrl Pts',(5.85520286590809,7.08209006146883,4.04313888631962));
#14591=CARTESIAN_POINT('Ctrl Pts',(5.84156747486463,7.07520486942886,4.12287606165967));
#14592=CARTESIAN_POINT('Ctrl Pts',(5.76326212603904,7.06138551553941,4.26551030037515));
#14593=CARTESIAN_POINT('Ctrl Pts',(5.58313571416996,7.04403789214147,4.37890493291776));
#14594=CARTESIAN_POINT('Ctrl Pts',(5.32733643620847,7.02308074340475,4.35047304239883));
#14595=CARTESIAN_POINT('Ctrl Pts',(5.14406551156473,7.00198204308889,4.16743848880527));
#14596=CARTESIAN_POINT('Ctrl Pts',(5.11430140308165,6.98073307206542,3.90823568037324));
#14597=CARTESIAN_POINT('Ctrl Pts',(5.2539756967838,6.9593299476571,3.68549505746316));
#14598=CARTESIAN_POINT('Ctrl Pts',(5.50385557975491,6.93776292440614,3.59765170680461));
#14599=CARTESIAN_POINT('Ctrl Pts',(5.746454002493,6.91683348560458,3.68233751904534));
#14600=CARTESIAN_POINT('Ctrl Pts',(5.88513081194609,6.89655721527044,3.8856066901103));
#14601=CARTESIAN_POINT('Ctrl Pts',(5.88561108039455,6.87695122617721,4.12342024789602));
#14602=CARTESIAN_POINT('Ctrl Pts',(5.7620912805646,6.85884906967209,4.30503249532845));
#14603=CARTESIAN_POINT('Ctrl Pts',(5.58439221890232,6.84228705858853,4.39044285766885));
#14604=CARTESIAN_POINT('Ctrl Pts',(5.43587731018536,6.82979711795253,4.39056857002489));
#14605=CARTESIAN_POINT('Ctrl Pts',(5.32531224002107,6.81976316059046,4.35179163381183));
#14606=CARTESIAN_POINT('Ctrl Pts',(5.22582219123238,6.80970122556429,4.28939485292107));
#14607=CARTESIAN_POINT('Ctrl Pts',(5.13200246986364,6.79707273454254,4.17202717151191));
#14608=CARTESIAN_POINT('Ctrl Pts',(5.09164094749547,6.78183341704652,3.99528331468449));
#14609=CARTESIAN_POINT('Ctrl Pts',(5.13200751743207,6.7665098094977,3.81754003421871));
#14610=CARTESIAN_POINT('Ctrl Pts',(5.24623575349236,6.75110199174121,3.67415956298011));
#14611=CARTESIAN_POINT('Ctrl Pts',(5.41224144571201,6.73560920651841,3.59409517730086));
#14612=CARTESIAN_POINT('Ctrl Pts',(5.59753307127925,6.72003176914412,3.59398376812156));
#14613=CARTESIAN_POINT('Ctrl Pts',(5.76552583542977,6.7043697251995,3.67473816518997));
#14614=CARTESIAN_POINT('Ctrl Pts',(5.88224637668914,6.68862335676344,3.82111570717619));
#14615=CARTESIAN_POINT('Ctrl Pts',(5.92933877872348,6.67103426452799,4.02514024338844));
#14616=CARTESIAN_POINT('Ctrl Pts',(5.85995562430613,6.65156702212541,4.25083041727868));
#14617=CARTESIAN_POINT('Ctrl Pts',(5.67407637808894,6.63196546184507,4.39925506328189));
#14618=CARTESIAN_POINT('Ctrl Pts',(5.50535216060145,6.61762539342909,4.42444600623728));
#14619=CARTESIAN_POINT('Ctrl Pts',(5.3605465743758,6.60503616153032,4.40267199067841));
#14620=CARTESIAN_POINT('Ctrl Pts',(5.22516696857318,6.59240538591147,4.33759897336023));
#14621=CARTESIAN_POINT('Ctrl Pts',(5.10399727465634,6.57608706132853,4.18587447130434));
#14622=CARTESIAN_POINT('Ctrl Pts',(5.06072881807943,6.55969079980481,3.9957755594979));
#14623=CARTESIAN_POINT('Ctrl Pts',(5.11111408899349,6.54047310824596,3.77281018900098));
#14624=CARTESIAN_POINT('Ctrl Pts',(5.30208506774464,6.51838444294906,3.58039325945438));
#14625=CARTESIAN_POINT('Ctrl Pts',(5.57344463256731,6.49615180944088,3.54987434760595));
#14626=CARTESIAN_POINT('Ctrl Pts',(5.76781931146614,6.47799290930932,3.64412456683428));
#14627=CARTESIAN_POINT('Ctrl Pts',(5.89995287193516,6.46117266087352,3.79146891932382));
#14628=CARTESIAN_POINT('Ctrl Pts',(5.95194793315776,6.44569200784306,3.97083844037072));
#14629=CARTESIAN_POINT('Ctrl Pts',(5.92101524437169,6.43015394352054,4.15103610674214));
#14630=CARTESIAN_POINT('Ctrl Pts',(5.82471537837473,6.41315680171824,4.32636138876989));
#14631=CARTESIAN_POINT('Ctrl Pts',(5.60334919178702,6.39182442975737,4.46603253787654));
#14632=CARTESIAN_POINT('Ctrl Pts',(5.28930632440049,6.36609845573924,4.43091101628552));
#14633=CARTESIAN_POINT('Ctrl Pts',(5.06476647708227,6.34025240232702,4.20670542372654));
#14634=CARTESIAN_POINT('Ctrl Pts',(5.02889907069948,6.3142971139968,3.89017648193371));
#14635=CARTESIAN_POINT('Ctrl Pts',(5.19901272516604,6.28823592961183,3.61906735374071));
#14636=CARTESIAN_POINT('Ctrl Pts',(5.50187330256082,6.26208782732235,3.51294889123812));
#14637=CARTESIAN_POINT('Ctrl Pts',(5.75522864687994,6.24022603278353,3.60140445329964));
#14638=CARTESIAN_POINT('Ctrl Pts',(5.8694004766967,6.22562326388648,3.72988152914194));
#14639=CARTESIAN_POINT('Ctrl Pts',(5.93521917425819,6.21393138166647,3.84871410099053));
#14640=CARTESIAN_POINT('Ctrl Pts',(5.9699545000092,6.2007640404577,4.00129391329599));
#14641=CARTESIAN_POINT('Ctrl Pts',(5.91603232645555,6.18025175472434,4.23954868417462));
#14642=CARTESIAN_POINT('Ctrl Pts',(5.75085163785764,6.16117154945629,4.40502717202795));
#14643=CARTESIAN_POINT('Ctrl Pts',(5.55107490688255,6.1435399111569,4.46192298098248));
#14644=CARTESIAN_POINT('Ctrl Pts',(5.37850386197236,6.12883720723606,4.45250910417445));
#14645=CARTESIAN_POINT('Ctrl Pts',(5.20506062246286,6.11265360212113,4.36891210542381));
#14646=CARTESIAN_POINT('Ctrl Pts',(5.07397022510475,6.09498817543275,4.20471986456681));
#14647=CARTESIAN_POINT('Ctrl Pts',(5.02724887723126,6.07731784476976,3.99979245739442));
#14648=CARTESIAN_POINT('Ctrl Pts',(5.07398000181797,6.05964215966279,3.79478075744986));
#14649=CARTESIAN_POINT('Ctrl Pts',(5.20512899117882,6.04196680287455,3.63051306675947));
#14650=CARTESIAN_POINT('Ctrl Pts',(5.39449791013073,6.02429430077605,3.53916197577409));
#14651=CARTESIAN_POINT('Ctrl Pts',(5.56957457418985,6.00957349714106,3.53928300415917));
#14652=CARTESIAN_POINT('Ctrl Pts',(5.68304311953453,5.99927347455427,3.57908441449588));
#14653=CARTESIAN_POINT('Ctrl Pts',(5.74286750570382,5.99338929587818,3.61214779557074));
#14654=CARTESIAN_POINT('Ctrl Pts',(5.82651752458846,5.98456439340875,3.67144751047707));
#14655=CARTESIAN_POINT('Ctrl Pts',(5.92457367352351,5.97133175061034,3.79451182749295));
#14656=CARTESIAN_POINT('Ctrl Pts',(5.97131861714195,5.95370439896441,3.99893579046224));
#14657=CARTESIAN_POINT('Ctrl Pts',(5.92459901326296,5.9360961851512,4.20307083437987));
#14658=CARTESIAN_POINT('Ctrl Pts',(5.80507236487523,5.91997636067228,4.35303796134367));
#14659=CARTESIAN_POINT('Ctrl Pts',(5.65434040611686,5.90534114871628,4.43611034923164));
#14660=CARTESIAN_POINT('Ctrl Pts',(5.45079337565466,5.88779962963185,4.47118188652743));
#14661=CARTESIAN_POINT('Ctrl Pts',(5.19748767042105,5.86591465359703,4.38257023322066));
#14662=CARTESIAN_POINT('Ctrl Pts',(5.0262253355364,5.83973026581737,4.1102456118929));
#14663=CARTESIAN_POINT('Ctrl Pts',(5.06249311301707,5.81363157422294,3.79188150756157));
#14664=CARTESIAN_POINT('Ctrl Pts',(5.28820296732657,5.78763167671582,3.56632359857709));
#14665=CARTESIAN_POINT('Ctrl Pts',(5.60433171174338,5.76173879777121,3.53092676719688));
#14666=CARTESIAN_POINT('Ctrl Pts',(5.8271423468097,5.74025670777543,3.67148617104396));
#14667=CARTESIAN_POINT('Ctrl Pts',(5.92424341235541,5.72313628975845,3.84810607771893));
#14668=CARTESIAN_POINT('Ctrl Pts',(5.94114425819813,5.71459769800728,3.94698841008634));
#14669=CARTESIAN_POINT('Ctrl Pts',(5.94115094957305,5.7103347709078,3.99658515196739));
#14670=CARTESIAN_POINT('Ctrl Pts',(5.8442633579502,7.03733205433023,3.99890364805841));
#14671=CARTESIAN_POINT('Ctrl Pts',(5.8442581197547,7.033994920285,4.03772931214518));
#14672=CARTESIAN_POINT('Ctrl Pts',(5.83104037018746,7.02733254813469,4.11486923947922));
#14673=CARTESIAN_POINT('Ctrl Pts',(5.75552618055734,7.01401654539893,4.25226823033117));
#14674=CARTESIAN_POINT('Ctrl Pts',(5.58280384378936,6.99739080062923,4.36069793188289));
#14675=CARTESIAN_POINT('Ctrl Pts',(5.33962002405483,6.97746235757696,4.33335540787856));
#14676=CARTESIAN_POINT('Ctrl Pts',(5.16682890132043,6.95754317780304,4.16039369672885));
#14677=CARTESIAN_POINT('Ctrl Pts',(5.13920853014916,6.93762223295465,3.91740209304229));
#14678=CARTESIAN_POINT('Ctrl Pts',(5.26947333563793,6.91768645343595,3.71016409897338));
#14679=CARTESIAN_POINT('Ctrl Pts',(5.50072401296219,6.89772870913039,3.62914290710299));
#14680=CARTESIAN_POINT('Ctrl Pts',(5.72372388246367,6.87847647854881,3.70723339336683));
#14681=CARTESIAN_POINT('Ctrl Pts',(5.85042194476176,6.85992603432529,3.89324231795015));
#14682=CARTESIAN_POINT('Ctrl Pts',(5.85070963937428,6.84207613283086,4.10972981319966));
#14683=CARTESIAN_POINT('Ctrl Pts',(5.73865422141122,6.82566665538221,4.27425669236962));
#14684=CARTESIAN_POINT('Ctrl Pts',(5.57815357745207,6.810706867649,4.35133307049917));
#14685=CARTESIAN_POINT('Ctrl Pts',(5.44441328362009,6.79945730366432,4.35140747521201));
#14686=CARTESIAN_POINT('Ctrl Pts',(5.34505646175606,6.79043938302152,4.31655337572742));
#14687=CARTESIAN_POINT('Ctrl Pts',(5.25576788953666,6.78140860275172,4.26054606594844));
#14688=CARTESIAN_POINT('Ctrl Pts',(5.1717433274605,6.77009209107834,4.15537468511295));
#14689=CARTESIAN_POINT('Ctrl Pts',(5.13570651291062,6.75647039032151,3.99739589300255));
#14690=CARTESIAN_POINT('Ctrl Pts',(5.17174572160623,6.74280160059864,3.83886918353745));
#14691=CARTESIAN_POINT('Ctrl Pts',(5.27346273046517,6.72908234649353,3.71124281622253));
#14692=CARTESIAN_POINT('Ctrl Pts',(5.42101179131082,6.71531148066912,3.6401110882049));
#14693=CARTESIAN_POINT('Ctrl Pts',(5.58544422096062,6.70148584866942,3.64003580689892));
#14694=CARTESIAN_POINT('Ctrl Pts',(5.73432346049268,6.68760313547377,3.71162565604183));
#14695=CARTESIAN_POINT('Ctrl Pts',(5.83764552929192,6.67366116797505,3.84122520535718));
#14696=CARTESIAN_POINT('Ctrl Pts',(5.87928444298638,6.658100912098,4.02169607449061));
#14697=CARTESIAN_POINT('Ctrl Pts',(5.81794296845177,6.64089543827006,4.22115320816706));
#14698=CARTESIAN_POINT('Ctrl Pts',(5.6537487144978,6.62358017931584,4.35224741413031));
#14699=CARTESIAN_POINT('Ctrl Pts',(5.50474573233506,6.61091566681907,4.37449449482154));
#14700=CARTESIAN_POINT('Ctrl Pts',(5.3768646872216,6.59979765360415,4.35526579110611));
#14701=CARTESIAN_POINT('Ctrl Pts',(5.25729954874086,6.58864209789496,4.29779828729648));
#14702=CARTESIAN_POINT('Ctrl Pts',(5.15025342040901,6.5742265315835,4.16377038217943));
#14703=CARTESIAN_POINT('Ctrl Pts',(5.11200030526049,6.55973534828414,3.99576364180229));
#14704=CARTESIAN_POINT('Ctrl Pts',(5.15654185679476,6.54274034280373,3.79858438441201));
#14705=CARTESIAN_POINT('Ctrl Pts',(5.32554784904026,6.52318707054893,3.62821328392619));
#14706=CARTESIAN_POINT('Ctrl Pts',(5.56613353860405,6.50347523010832,3.60107938902761));
#14707=CARTESIAN_POINT('Ctrl Pts',(5.73877029295882,6.48734943548394,3.68475125508372));
#14708=CARTESIAN_POINT('Ctrl Pts',(5.85627571304628,6.47239252636156,3.81575918380156));
#14709=CARTESIAN_POINT('Ctrl Pts',(5.90263031720046,6.45860635937458,3.97548974074165));
#14710=CARTESIAN_POINT('Ctrl Pts',(5.87505167436944,6.44474372928567,4.13626778107872));
#14711=CARTESIAN_POINT('Ctrl Pts',(5.78903514141083,6.42955803390157,4.29291835106576));
#14712=CARTESIAN_POINT('Ctrl Pts',(5.59088448553645,6.41045798350198,4.41808744129809));
#14713=CARTESIAN_POINT('Ctrl Pts',(5.30873518287549,6.38734750124527,4.38670311299745));
#14714=CARTESIAN_POINT('Ctrl Pts',(5.10615471140587,6.36404684857898,4.18468451257222));
#14715=CARTESIAN_POINT('Ctrl Pts',(5.07349898841052,6.34055522359989,3.8982098092804));
#14716=CARTESIAN_POINT('Ctrl Pts',(5.22791505782553,6.31687679944705,3.65170107095422));
#14717=CARTESIAN_POINT('Ctrl Pts',(5.50431592493739,6.29300768975538,3.55461983394832));
#14718=CARTESIAN_POINT('Ctrl Pts',(5.73671787489177,6.27296418176745,3.6355503842994));
#14719=CARTESIAN_POINT('Ctrl Pts',(5.84183688606317,6.25952452604128,3.75378707156832));
#14720=CARTESIAN_POINT('Ctrl Pts',(5.90252063540586,6.24874582138889,3.86334104486593));
#14721=CARTESIAN_POINT('Ctrl Pts',(5.93466081634591,6.23658242737163,4.00429106496237));
#14722=CARTESIAN_POINT('Ctrl Pts',(5.88477257211492,6.21756897840495,4.22516592599398));
#14723=CARTESIAN_POINT('Ctrl Pts',(5.73112374226898,6.19980983242131,4.37935499119927));
#14724=CARTESIAN_POINT('Ctrl Pts',(5.54437866031431,6.18333055162171,4.43259622705531));
#14725=CARTESIAN_POINT('Ctrl Pts',(5.38261999067874,6.16955106486449,4.42380810286847));
#14726=CARTESIAN_POINT('Ctrl Pts',(5.21948440418905,6.15433461785036,4.34526151688322));
#14727=CARTESIAN_POINT('Ctrl Pts',(5.09567527200945,6.13766356859339,4.19033418142023));
#14728=CARTESIAN_POINT('Ctrl Pts',(5.05132292060661,6.120920804985,3.99616808757238));
#14729=CARTESIAN_POINT('Ctrl Pts',(5.09568013075446,6.10411152452373,3.80114024004156));
#14730=CARTESIAN_POINT('Ctrl Pts',(5.2208564304236,6.08723548924311,3.64421655461967));
#14731=CARTESIAN_POINT('Ctrl Pts',(5.40236843774688,6.07029554676657,3.55655082292256));
#14732=CARTESIAN_POINT('Ctrl Pts',(5.57090761649076,6.05612632794669,3.55659431162632));
#14733=CARTESIAN_POINT('Ctrl Pts',(5.68047831247714,6.04618144828711,3.59501288603736));
#14734=CARTESIAN_POINT('Ctrl Pts',(5.7383337836807,6.04049119521234,3.62698653839934));
#14735=CARTESIAN_POINT('Ctrl Pts',(5.8193132044321,6.03194870990487,3.68438770351889));
#14736=CARTESIAN_POINT('Ctrl Pts',(5.91452854847537,6.0191093147926,3.80377513400947));
#14737=CARTESIAN_POINT('Ctrl Pts',(5.96017726931528,6.00193511332281,4.00295549686061));
#14738=CARTESIAN_POINT('Ctrl Pts',(5.91454763656368,5.98470857921717,4.2027269727812));
#14739=CARTESIAN_POINT('Ctrl Pts',(5.79716877045588,5.96887147306035,4.35014107428084));
#14740=CARTESIAN_POINT('Ctrl Pts',(5.64852424861931,5.95443918265348,4.43210799719531));
#14741=CARTESIAN_POINT('Ctrl Pts',(5.44716731617039,5.93708678955292,4.46686180108763));
#14742=CARTESIAN_POINT('Ctrl Pts',(5.19528800450862,5.91533634052886,4.37903445531321));
#14743=CARTESIAN_POINT('Ctrl Pts',(5.02367424394978,5.88914912040216,4.10682213449717));
#14744=CARTESIAN_POINT('Ctrl Pts',(5.05983407646609,5.86288698339694,3.78630359033442));
#14745=CARTESIAN_POINT('Ctrl Pts',(5.28822019826199,5.83655644865667,3.55758071132317));
#14746=CARTESIAN_POINT('Ctrl Pts',(5.61042287602758,5.81016939852405,3.52114893229972));
#14747=CARTESIAN_POINT('Ctrl Pts',(5.83908979198061,5.78814211888601,3.66511277419047));
#14748=CARTESIAN_POINT('Ctrl Pts',(5.93920546082742,5.77050202961558,3.8470873725861));
#14749=CARTESIAN_POINT('Ctrl Pts',(5.95669478049843,5.76167432127745,3.94932370527045));
#14750=CARTESIAN_POINT('Ctrl Pts',(5.95670170074323,5.75726558623602,4.00061683995683));
#14751=CARTESIAN_POINT('Ctrl Pts',(5.87514548417672,6.99854044864851,3.99557360787966));
#14752=CARTESIAN_POINT('Ctrl Pts',(5.87513978765661,6.99491132651841,4.03779638791872));
#14753=CARTESIAN_POINT('Ctrl Pts',(5.86075022359954,6.98766329031147,4.12172125899622));
#14754=CARTESIAN_POINT('Ctrl Pts',(5.77883107645889,6.97322759641233,4.27068148293984));
#14755=CARTESIAN_POINT('Ctrl Pts',(5.59230633485985,6.95528685852212,4.38753321295925));
#14756=CARTESIAN_POINT('Ctrl Pts',(5.33155020564179,6.93391865832403,4.35791618403263));
#14757=CARTESIAN_POINT('Ctrl Pts',(5.14773246729608,6.91270540416619,4.17347705756876));
#14758=CARTESIAN_POINT('Ctrl Pts',(5.11883580759173,6.89164103056227,3.9164440087751));
#14759=CARTESIAN_POINT('Ctrl Pts',(5.25588116695966,6.87071957668565,3.6990566497247));
#14760=CARTESIAN_POINT('Ctrl Pts',(5.49694403853312,6.84993083868618,3.6149532499762));
#14761=CARTESIAN_POINT('Ctrl Pts',(5.72739217434572,6.83003349550605,3.69599197049964));
#14762=CARTESIAN_POINT('Ctrl Pts',(5.85719964701457,6.81100327064808,3.88700464630704));
#14763=CARTESIAN_POINT('Ctrl Pts',(5.85726081296606,6.79281909841024,4.10758802917809));
#14764=CARTESIAN_POINT('Ctrl Pts',(5.74373291807669,6.77622423972196,4.27389444303247));
#14765=CARTESIAN_POINT('Ctrl Pts',(5.58236852338651,6.76119137058875,4.35125834030399));
#14766=CARTESIAN_POINT('Ctrl Pts',(5.44867419960033,6.74994884661536,4.35125385557247));
#14767=CARTESIAN_POINT('Ctrl Pts',(5.34976030800238,6.74097144095651,4.31653614511533));
#14768=CARTESIAN_POINT('Ctrl Pts',(5.26110773818199,6.73200480430205,4.26090950185114));
#14769=CARTESIAN_POINT('Ctrl Pts',(5.17808610936031,6.72081958457785,4.15686365468362));
#14770=CARTESIAN_POINT('Ctrl Pts',(5.1427384642525,6.70742370332015,4.00146629817937));
#14771=CARTESIAN_POINT('Ctrl Pts',(5.17808628986628,6.69405440549435,3.84640454479009));
#14772=CARTESIAN_POINT('Ctrl Pts',(5.27713337356397,6.68070956969354,3.72228233330786));
#14773=CARTESIAN_POINT('Ctrl Pts',(5.41998780176605,6.66738391686113,3.6535162350639));
#14774=CARTESIAN_POINT('Ctrl Pts',(5.57831764719913,6.65407511732755,3.65353579167895));
#14775=CARTESIAN_POINT('Ctrl Pts',(5.72089719398017,6.64077986955346,3.72219848416115));
#14776=CARTESIAN_POINT('Ctrl Pts',(5.81930953143935,6.62749439614206,3.84577722805825));
#14777=CARTESIAN_POINT('Ctrl Pts',(5.85870394850306,6.61274185884821,4.01697267297566));
#14778=CARTESIAN_POINT('Ctrl Pts',(5.80067105304151,6.59651509694839,4.20503754829806));
#14779=CARTESIAN_POINT('Ctrl Pts',(5.64666780825017,6.58028993315573,4.32776333798744));
#14780=CARTESIAN_POINT('Ctrl Pts',(5.50774076906622,6.56848394985099,4.34843470371925));
#14781=CARTESIAN_POINT('Ctrl Pts',(5.38885142963878,6.55814860077465,4.33055181655375));
#14782=CARTESIAN_POINT('Ctrl Pts',(5.27804026744975,6.54780951370302,4.2772266172093));
#14783=CARTESIAN_POINT('Ctrl Pts',(5.17927293647025,6.53450161770272,4.15344678062057));
#14784=CARTESIAN_POINT('Ctrl Pts',(5.14416812305239,6.52118046944049,3.99895936753469));
#14785=CARTESIAN_POINT('Ctrl Pts',(5.1850453990095,6.50561478324366,3.81835726355173));
#14786=CARTESIAN_POINT('Ctrl Pts',(5.339284997864,6.48779307370435,3.66315400412196));
#14787=CARTESIAN_POINT('Ctrl Pts',(5.55754831918104,6.46991368775191,3.63872503876236));
#14788=CARTESIAN_POINT('Ctrl Pts',(5.71350848036609,6.45534555587482,3.71438173891507));
#14789=CARTESIAN_POINT('Ctrl Pts',(5.81940093081938,6.44186425747974,3.83248890666509));
#14790=CARTESIAN_POINT('Ctrl Pts',(5.86099636209716,6.42947631893566,3.97607363283317));
#14791=CARTESIAN_POINT('Ctrl Pts',(5.83624924861445,6.41704875670862,4.12020838390855));
#14792=CARTESIAN_POINT('Ctrl Pts',(5.75924576580022,6.40345957109736,4.26039065665031));
#14793=CARTESIAN_POINT('Ctrl Pts',(5.58230732141824,6.38641243046477,4.37202924255808));
#14794=CARTESIAN_POINT('Ctrl Pts',(5.33119627254454,6.36584482021927,4.34397642119019));
#14795=CARTESIAN_POINT('Ctrl Pts',(5.15140636995601,6.34515949086949,4.16454562210437));
#14796=CARTESIAN_POINT('Ctrl Pts',(5.12254982607975,6.32434519787953,3.91070033361363));
#14797=CARTESIAN_POINT('Ctrl Pts',(5.25920873518247,6.30340142939672,3.6926602572414));
#14798=CARTESIAN_POINT('Ctrl Pts',(5.50347393537872,6.28230883810381,3.60690759285009));
#14799=CARTESIAN_POINT('Ctrl Pts',(5.70869616727121,6.26461043075207,3.67839455761512));
#14800=CARTESIAN_POINT('Ctrl Pts',(5.80150749996396,6.2527445027482,3.78278841553677));
#14801=CARTESIAN_POINT('Ctrl Pts',(5.8550859977429,6.24322788838423,3.87951569410302));
#14802=CARTESIAN_POINT('Ctrl Pts',(5.88346434910103,6.23248866320778,4.00396460760673));
#14803=CARTESIAN_POINT('Ctrl Pts',(5.83941409539019,6.21569758858433,4.19902206859976));
#14804=CARTESIAN_POINT('Ctrl Pts',(5.70367326626789,6.20000650214883,4.33527098884019));
#14805=CARTESIAN_POINT('Ctrl Pts',(5.53855228655731,6.18543517970738,4.38235651612384));
#14806=CARTESIAN_POINT('Ctrl Pts',(5.39543801792977,6.17324367379672,4.37458667586454));
#14807=CARTESIAN_POINT('Ctrl Pts',(5.25098024432611,6.15976998349194,4.30505194274034));
#14808=CARTESIAN_POINT('Ctrl Pts',(5.14121655731439,6.14499160555445,4.16773264727778));
#14809=CARTESIAN_POINT('Ctrl Pts',(5.10182587914745,6.13013154458964,3.99540643427926));
#14810=CARTESIAN_POINT('Ctrl Pts',(5.14122514831917,6.11519028373789,3.8220564397272));
#14811=CARTESIAN_POINT('Ctrl Pts',(5.25263588248017,6.10016628060021,3.68233820392778));
#14812=CARTESIAN_POINT('Ctrl Pts',(5.41448657988468,6.08505886588137,3.60412985666001));
#14813=CARTESIAN_POINT('Ctrl Pts',(5.56506704731687,6.07239919129658,3.60413578617919));
#14814=CARTESIAN_POINT('Ctrl Pts',(5.66311283101293,6.06350038653797,3.63850704060478));
#14815=CARTESIAN_POINT('Ctrl Pts',(5.7149221186375,6.05840477958295,3.66713842572877));
#14816=CARTESIAN_POINT('Ctrl Pts',(5.78747702938897,6.05075080923013,3.7185669337241));
#14817=CARTESIAN_POINT('Ctrl Pts',(5.87293025946013,6.03923050065618,3.82566146039982));
#14818=CARTESIAN_POINT('Ctrl Pts',(5.91402507704787,6.02378513403553,4.00476477146208));
#14819=CARTESIAN_POINT('Ctrl Pts',(5.87294369145138,6.00825508165675,4.18486099195512));
#14820=CARTESIAN_POINT('Ctrl Pts',(5.76690353827561,5.99394133612039,4.31811566915106));
#14821=CARTESIAN_POINT('Ctrl Pts',(5.63226512122908,5.98086723592559,4.39238906025841));
#14822=CARTESIAN_POINT('Ctrl Pts',(5.44950474947794,5.96511502927026,4.42397005765718));
#14823=CARTESIAN_POINT('Ctrl Pts',(5.22008211053465,5.94530667428613,4.34415650242552));
#14824=CARTESIAN_POINT('Ctrl Pts',(5.06291182507567,5.92134913814384,4.09528547532897));
#14825=CARTESIAN_POINT('Ctrl Pts',(5.09590900327192,5.89720669469332,3.80066624542902));
#14826=CARTESIAN_POINT('Ctrl Pts',(5.30668586808294,5.87288210191658,3.58923668118618));
#14827=CARTESIAN_POINT('Ctrl Pts',(5.60579413240307,5.84838086936144,3.55513713761874));
#14828=CARTESIAN_POINT('Ctrl Pts',(5.81936747109835,5.82781552400804,3.68933059315267));
#14829=CARTESIAN_POINT('Ctrl Pts',(5.91324358998992,5.81128381242343,3.85984598368901));
#14830=CARTESIAN_POINT('Ctrl Pts',(5.92970378689351,5.80298590584205,3.95593351696052));
#14831=CARTESIAN_POINT('Ctrl Pts',(5.92971029794461,5.79883785906193,4.00419369140481));
#14832=CARTESIAN_POINT('Ctrl Pts',(5.92479734822298,6.99869271407564,3.99559339418157));
#14833=CARTESIAN_POINT('Ctrl Pts',(5.92479090997151,6.99459105192559,4.04331390965279));
#14834=CARTESIAN_POINT('Ctrl Pts',(5.90850975380561,6.98638756199577,4.1382994503635));
#14835=CARTESIAN_POINT('Ctrl Pts',(5.8157856671956,6.97004679073908,4.30691427794729));
#14836=CARTESIAN_POINT('Ctrl Pts',(5.60456312519679,6.94972761837475,4.43926282438681));
#14837=CARTESIAN_POINT('Ctrl Pts',(5.30924514470025,6.92552625657262,4.40571412404912));
#14838=CARTESIAN_POINT('Ctrl Pts',(5.10115155224644,6.90150776708021,4.19688142095042));
#14839=CARTESIAN_POINT('Ctrl Pts',(5.06851049643939,6.87767566403273,3.90609185048507));
#14840=CARTESIAN_POINT('Ctrl Pts',(5.22342892068834,6.85403159761471,3.66049532779896));
#14841=CARTESIAN_POINT('Ctrl Pts',(5.49540131761851,6.8305770702376,3.56571109549459));
#14842=CARTESIAN_POINT('Ctrl Pts',(5.75478373950727,6.80817442310058,3.65704418598113));
#14843=CARTESIAN_POINT('Ctrl Pts',(5.90047506910969,6.78680000659775,3.8716090579534));
#14844=CARTESIAN_POINT('Ctrl Pts',(5.90043765469484,6.76643101559881,4.11867588537419));
#14845=CARTESIAN_POINT('Ctrl Pts',(5.77356623131722,6.7478962216523,4.30433440185149));
#14846=CARTESIAN_POINT('Ctrl Pts',(5.59386479707093,6.73115456608272,4.39041942156343));
#14847=CARTESIAN_POINT('Ctrl Pts',(5.44539655895096,6.71866722776999,4.39036886564142));
#14848=CARTESIAN_POINT('Ctrl Pts',(5.33579942713953,6.70871882259051,4.35189016716179));
#14849=CARTESIAN_POINT('Ctrl Pts',(5.23771902383275,6.69879786668875,4.2903366305777));
#14850=CARTESIAN_POINT('Ctrl Pts',(5.14611136868914,6.686446054238,4.17544171847082));
#14851=CARTESIAN_POINT('Ctrl Pts',(5.10728479879167,6.67170559659797,4.00445121458595));
#14852=CARTESIAN_POINT('Ctrl Pts',(5.14611211950831,6.65704405744421,3.83444276345394));
#14853=CARTESIAN_POINT('Ctrl Pts',(5.25438505285132,6.64245966977581,3.69887894687364));
#14854=CARTESIAN_POINT('Ctrl Pts',(5.40990166233343,6.62795227611534,3.62410389391192));
#14855=CARTESIAN_POINT('Ctrl Pts',(5.5815496819327,6.61351997914256,3.62420401324371));
#14856=CARTESIAN_POINT('Ctrl Pts',(5.73544946394382,6.59916119992895,3.69841415911542));
#14857=CARTESIAN_POINT('Ctrl Pts',(5.84118479017196,6.58487472963496,3.83131690200048));
#14858=CARTESIAN_POINT('Ctrl Pts',(5.88325122365517,6.56907782799123,4.01459123943289));
#14859=CARTESIAN_POINT('Ctrl Pts',(5.82128683856772,6.55180183670017,4.21474716794292));
#14860=CARTESIAN_POINT('Ctrl Pts',(5.65822534686918,6.53463077872286,4.34442789266045));
#14861=CARTESIAN_POINT('Ctrl Pts',(5.51207474544734,6.52220844326274,4.36609029268673));
#14862=CARTESIAN_POINT('Ctrl Pts',(5.38742554303644,6.51137100417828,4.34733263783343));
#14863=CARTESIAN_POINT('Ctrl Pts',(5.27165764889733,6.50056364797766,4.2915430638631));
#14864=CARTESIAN_POINT('Ctrl Pts',(5.16905588565897,6.48672787446753,4.16279863377245));
#14865=CARTESIAN_POINT('Ctrl Pts',(5.13283917983621,6.47294482309939,4.00299700475136));
#14866=CARTESIAN_POINT('Ctrl Pts',(5.1750114352257,6.45692788066795,3.81720051065741));
#14867=CARTESIAN_POINT('Ctrl Pts',(5.33289108133986,6.43870149704958,3.65876416560081));
#14868=CARTESIAN_POINT('Ctrl Pts',(5.55419693287486,6.42057082795549,3.63430277213249));
#14869=CARTESIAN_POINT('Ctrl Pts',(5.71118304201485,6.40589452371311,3.71057513225082));
#14870=CARTESIAN_POINT('Ctrl Pts',(5.81726355608341,6.39238507064568,3.82897080987877));
#14871=CARTESIAN_POINT('Ctrl Pts',(5.85858981339439,6.38003097260466,3.97213930596044));
#14872=CARTESIAN_POINT('Ctrl Pts',(5.83401059568513,6.36771004387122,4.11499949089278));
#14873=CARTESIAN_POINT('Ctrl Pts',(5.75793177724685,6.35429201109606,4.25337987346692));
#14874=CARTESIAN_POINT('Ctrl Pts',(5.5841434597572,6.33755678598937,4.36270673919398));
#14875=CARTESIAN_POINT('Ctrl Pts',(5.33972856653595,6.31752970311076,4.33506481527608));
#14876=CARTESIAN_POINT('Ctrl Pts',(5.16631525257735,6.29754423858894,4.16154035829682));
#14877=CARTESIAN_POINT('Ctrl Pts',(5.1389670014894,6.27759361927993,3.91823011012584));
#14878=CARTESIAN_POINT('Ctrl Pts',(5.26923427006138,6.25765586167643,3.71098251993868));
#14879=CARTESIAN_POINT('Ctrl Pts',(5.49997414943137,6.2377376533677,3.63028623162157));
#14880=CARTESIAN_POINT('Ctrl Pts',(5.69234045845551,6.2211328327069,3.69754386482986));
#14881=CARTESIAN_POINT('Ctrl Pts',(5.77889109313146,6.21006107345164,3.79495147685565));
#14882=CARTESIAN_POINT('Ctrl Pts',(5.8287628675858,6.20120152181681,3.88499526513206));
#14883=CARTESIAN_POINT('Ctrl Pts',(5.85505659115829,6.1912298978419,4.00053965484459));
#14884=CARTESIAN_POINT('Ctrl Pts',(5.81423820297505,6.17570552245903,4.18084805030103));
#14885=CARTESIAN_POINT('Ctrl Pts',(5.68925420776868,6.16126646712905,4.3060653674419));
#14886=CARTESIAN_POINT('Ctrl Pts',(5.53801582331833,6.14791748162507,4.34914806893716));
#14887=CARTESIAN_POINT('Ctrl Pts',(5.40729475179393,6.13677964483745,4.34202352685408));
#14888=CARTESIAN_POINT('Ctrl Pts',(5.27577798314163,6.12450821845862,4.27866007683168));
#14889=CARTESIAN_POINT('Ctrl Pts',(5.17621152498865,6.11109298436855,4.15400034396759));
#14890=CARTESIAN_POINT('Ctrl Pts',(5.14062815757453,6.09764920528476,3.99810258706931));
#14891=CARTESIAN_POINT('Ctrl Pts',(5.17621864961869,6.08416957526783,3.84175996625641));
#14892=CARTESIAN_POINT('Ctrl Pts',(5.27645693346059,6.07065378662253,3.71612247842351));
#14893=CARTESIAN_POINT('Ctrl Pts',(5.4216736508846,6.05709829175107,3.64600249711584));
#14894=CARTESIAN_POINT('Ctrl Pts',(5.55642697968229,6.04576775227701,3.64603929507313));
#14895=CARTESIAN_POINT('Ctrl Pts',(5.6440193761318,6.03781700092045,3.67675205629796));
#14896=CARTESIAN_POINT('Ctrl Pts',(5.69026902046296,6.03326803369609,3.70231145507745));
#14897=CARTESIAN_POINT('Ctrl Pts',(5.75500475915597,6.02643854964378,3.74819976516779));
#14898=CARTESIAN_POINT('Ctrl Pts',(5.83113812206107,6.01617049150737,3.84365344915576));
#14899=CARTESIAN_POINT('Ctrl Pts',(5.86766196956311,6.00242939725551,4.00298279625502));
#14900=CARTESIAN_POINT('Ctrl Pts',(5.8311547471775,5.98863491997195,4.16292338324265));
#14901=CARTESIAN_POINT('Ctrl Pts',(5.73709557243115,5.97593951486642,4.28108823702175));
#14902=CARTESIAN_POINT('Ctrl Pts',(5.61781643785115,5.96435631741718,4.34688070547426));
#14903=CARTESIAN_POINT('Ctrl Pts',(5.45603306860374,5.95041149725462,4.37482578814888));
#14904=CARTESIAN_POINT('Ctrl Pts',(5.25316590304169,5.93289348529237,4.30421133407663));
#14905=CARTESIAN_POINT('Ctrl Pts',(5.114334341813,5.91172572229907,4.08431983563909));
#14906=CARTESIAN_POINT('Ctrl Pts',(5.14347742913921,5.89040379142845,3.82415207297242));
#14907=CARTESIAN_POINT('Ctrl Pts',(5.32958757437269,5.8689234097876,3.63744549574417));
#14908=CARTESIAN_POINT('Ctrl Pts',(5.593792158646,5.84727920751737,3.60729146399766));
#14909=CARTESIAN_POINT('Ctrl Pts',(5.78261609629093,5.82909825547531,3.72587469920206));
#14910=CARTESIAN_POINT('Ctrl Pts',(5.86569002809564,5.81446997132799,3.87675017989571));
#14911=CARTESIAN_POINT('Ctrl Pts',(5.88026841209617,5.80712385602455,3.96181257456008));
#14912=CARTESIAN_POINT('Ctrl Pts',(5.88027418431338,5.80344650399414,4.00459648223716));
#14913=CARTESIAN_POINT('Ctrl Pts',(5.95590306687186,7.03727919710367,3.99891416684745));
#14914=CARTESIAN_POINT('Ctrl Pts',(5.95589616141154,7.03287988693566,4.05009764838621));
#14915=CARTESIAN_POINT('Ctrl Pts',(5.93842634741758,7.02407009585036,4.15210152738218));
#14916=CARTESIAN_POINT('Ctrl Pts',(5.83862476994702,7.00647265914313,4.33368324484612));
#14917=CARTESIAN_POINT('Ctrl Pts',(5.61038748339536,6.98450279632803,4.47695533665323));
#14918=CARTESIAN_POINT('Ctrl Pts',(5.28951816532253,6.95820805223714,4.44078048995406));
#14919=CARTESIAN_POINT('Ctrl Pts',(5.06216227665699,6.931985960868,4.21299691146494));
#14920=CARTESIAN_POINT('Ctrl Pts',(5.02611958609637,6.90584826166672,3.89414010003615));
#14921=CARTESIAN_POINT('Ctrl Pts',(5.19653980841186,6.87980141769972,3.62350837417727));
#14922=CARTESIAN_POINT('Ctrl Pts',(5.49724448642999,6.85385971296279,3.5184785366482));
#14923=CARTESIAN_POINT('Ctrl Pts',(5.78525918241898,6.82898632949769,3.61969120955249));
#14924=CARTESIAN_POINT('Ctrl Pts',(5.94765088502646,6.80517631696329,3.85861234902237));
#14925=CARTESIAN_POINT('Ctrl Pts',(5.94772393662232,6.7824215728438,4.1346057376524));
#14926=CARTESIAN_POINT('Ctrl Pts',(5.8057000315009,6.76166065837722,4.34261111889119));
#14927=CARTESIAN_POINT('Ctrl Pts',(5.60401485141267,6.74286906514136,4.4392793038978));
#14928=CARTESIAN_POINT('Ctrl Pts',(5.43709628111368,6.72882975921881,4.43925283529324));
#14929=CARTESIAN_POINT('Ctrl Pts',(5.3137380044414,6.71763253999929,4.39594951157785));
#14930=CARTESIAN_POINT('Ctrl Pts',(5.20326509995367,6.70645831516364,4.32662502497686));
#14931=CARTESIAN_POINT('Ctrl Pts',(5.09996040114962,6.69253290488073,4.19710330322307));
#14932=CARTESIAN_POINT('Ctrl Pts',(5.05610887744417,6.67589443882275,4.0040968779241));
#14933=CARTESIAN_POINT('Ctrl Pts',(5.09995854584184,6.65932883970079,3.8119966041178));
#14934=CARTESIAN_POINT('Ctrl Pts',(5.22238370498492,6.64283754317385,3.65868097433416));
#14935=CARTESIAN_POINT('Ctrl Pts',(5.39835972294708,6.62642245590569,3.57405122274256));
#14936=CARTESIAN_POINT('Ctrl Pts',(5.59268901758044,6.61008477200057,3.57415252520102));
#14937=CARTESIAN_POINT('Ctrl Pts',(5.7669805856365,6.5938259218282,3.6581859819855));
#14938=CARTESIAN_POINT('Ctrl Pts',(5.88673791828364,6.57764687866966,3.80870886087705));
#14939=CARTESIAN_POINT('Ctrl Pts',(5.93438063104257,6.55976041103417,4.01626669154502));
#14940=CARTESIAN_POINT('Ctrl Pts',(5.8642069662864,6.54020125406153,4.24287570953169));
#14941=CARTESIAN_POINT('Ctrl Pts',(5.6797098229945,6.520777947123,4.3895696010608));
#14942=CARTESIAN_POINT('Ctrl Pts',(5.51451149302123,6.50673855146733,4.41403838239402));
#14943=CARTESIAN_POINT('Ctrl Pts',(5.37370646222636,6.49449746275024,4.39284888630218));
#14944=CARTESIAN_POINT('Ctrl Pts',(5.24303700980646,6.48230054675382,4.32985873556225));
#14945=CARTESIAN_POINT('Ctrl Pts',(5.12738220646008,6.46670249550793,4.18469192949528));
#14946=CARTESIAN_POINT('Ctrl Pts',(5.08664089228909,6.4511905915314,4.00479453396285));
#14947=CARTESIAN_POINT('Ctrl Pts',(5.13407589369759,6.43319124323249,3.7959812029093));
#14948=CARTESIAN_POINT('Ctrl Pts',(5.31118286959745,6.41276495133761,3.61841802211263));
#14949=CARTESIAN_POINT('Ctrl Pts',(5.55853958666605,6.39250501417649,3.59122528508859));
#14950=CARTESIAN_POINT('Ctrl Pts',(5.73342093935756,6.37615866441498,3.67625437042241));
#14951=CARTESIAN_POINT('Ctrl Pts',(5.85133313713545,6.36113952640084,3.80790529683591));
#14952=CARTESIAN_POINT('Ctrl Pts',(5.89706702481703,6.34745121016953,3.96663113427204));
#14953=CARTESIAN_POINT('Ctrl Pts',(5.86987038418826,6.33383538334179,4.12451552814598));
#14954=CARTESIAN_POINT('Ctrl Pts',(5.78594882016984,6.31904256295841,4.27708653025637));
#14955=CARTESIAN_POINT('Ctrl Pts',(5.59494613134684,6.30066694840301,4.39701695335078));
#14956=CARTESIAN_POINT('Ctrl Pts',(5.32792628430838,6.2787914117074,4.36655869826738));
#14957=CARTESIAN_POINT('Ctrl Pts',(5.13973148170606,6.25708954605818,4.17786422412083));
#14958=CARTESIAN_POINT('Ctrl Pts',(5.11048151266317,6.23555198387054,3.91512091298944));
#14959=CARTESIAN_POINT('Ctrl Pts',(5.25045794049214,6.21418524204142,3.69297296555494));
#14960=CARTESIAN_POINT('Ctrl Pts',(5.49641917714145,6.19296358963855,3.60727428386931));
#14961=CARTESIAN_POINT('Ctrl Pts',(5.69983988901561,6.17540944769186,3.67867241225569));
#14962=CARTESIAN_POINT('Ctrl Pts',(5.79086497922878,6.16376212897976,3.78118818554554));
#14963=CARTESIAN_POINT('Ctrl Pts',(5.84321117645942,6.15446420449365,3.87570466796909));
#14964=CARTESIAN_POINT('Ctrl Pts',(5.87065814437396,6.14403327021692,3.99661498745638));
#14965=CARTESIAN_POINT('Ctrl Pts',(5.82805008788353,6.12787459541677,4.18430575396648));
#14966=CARTESIAN_POINT('Ctrl Pts',(5.69862866856204,6.11295020903452,4.31365122027558));
#14967=CARTESIAN_POINT('Ctrl Pts',(5.54313378493208,6.0992304546001,4.35787902005905));
#14968=CARTESIAN_POINT('Ctrl Pts',(5.40926178871448,6.08782855308313,4.35054539341534));
#14969=CARTESIAN_POINT('Ctrl Pts',(5.27525709486542,6.07532528539318,4.28587506508975));
#14970=CARTESIAN_POINT('Ctrl Pts',(5.17439041177087,6.06173195224338,4.15944267362621));
#14971=CARTESIAN_POINT('Ctrl Pts',(5.13861259214682,6.04817811425488,4.00222176271348));
#14972=CARTESIAN_POINT('Ctrl Pts',(5.17439053825513,6.03466753046012,3.84546673219833));
#14973=CARTESIAN_POINT('Ctrl Pts',(5.27444029713,6.0211930273313,3.72023060681213));
#14974=CARTESIAN_POINT('Ctrl Pts',(5.41852484284517,6.00775286378202,3.65076614242221));
#14975=CARTESIAN_POINT('Ctrl Pts',(5.55146977058118,5.99657679058691,3.65088710095702));
#14976=CARTESIAN_POINT('Ctrl Pts',(5.63753376629596,5.98876512785074,3.68107859235753));
#14977=CARTESIAN_POINT('Ctrl Pts',(5.68288882480457,5.98430436242261,3.70614602139524));
#14978=CARTESIAN_POINT('Ctrl Pts',(5.74628736488937,5.97761664176628,3.75108884668273));
#14979=CARTESIAN_POINT('Ctrl Pts',(5.82053438649198,5.96759894686408,3.84429050484334));
#14980=CARTESIAN_POINT('Ctrl Pts',(5.8559045113389,5.9542634039028,3.9989889909768));
#14981=CARTESIAN_POINT('Ctrl Pts',(5.82055051327847,5.94094654736442,4.15342083439052));
#14982=CARTESIAN_POINT('Ctrl Pts',(5.7301138579932,5.92875253598539,4.2668953204214));
#14983=CARTESIAN_POINT('Ctrl Pts',(5.61600089164756,5.91767493945766,4.32978774586891));
#14984=CARTESIAN_POINT('Ctrl Pts',(5.46180933263781,5.90438928265866,4.35636097149178));
#14985=CARTESIAN_POINT('Ctrl Pts',(5.26964185338532,5.88779310902171,4.28920833470193));
#14986=CARTESIAN_POINT('Ctrl Pts',(5.13926593838416,5.86788359492209,4.0821491463144));
#14987=CARTESIAN_POINT('Ctrl Pts',(5.1667763249041,5.84797174518985,3.83909164331259));
#14988=CARTESIAN_POINT('Ctrl Pts',(5.33971434420192,5.82804129686562,3.66595696613271));
#14989=CARTESIAN_POINT('Ctrl Pts',(5.58345731087934,5.8080821094971,3.63840397287366));
#14990=CARTESIAN_POINT('Ctrl Pts',(5.75648703078364,5.79142038910681,3.74728751079694));
#14991=CARTESIAN_POINT('Ctrl Pts',(5.83232118693006,5.77805963303851,3.88511710631332));
#14992=CARTESIAN_POINT('Ctrl Pts',(5.84558001546802,5.77137200360298,3.96257247922028));
#14993=CARTESIAN_POINT('Ctrl Pts',(5.8455852749944,5.76802127557217,4.00155630169246));
#14994=CARTESIAN_POINT('Ctrl Pts',(5.94467745847827,7.085541872266,4.00306091406361));
#14995=CARTESIAN_POINT('Ctrl Pts',(5.94467071320255,7.08124461202357,4.05305710253085));
#14996=CARTESIAN_POINT('Ctrl Pts',(5.92762764874893,7.07263818921979,4.15272355020168));
#14997=CARTESIAN_POINT('Ctrl Pts',(5.82985601806925,7.05538712363623,4.33077138583792));
#14998=CARTESIAN_POINT('Ctrl Pts',(5.60523592604193,7.03375625002402,4.47208979961085));
#14999=CARTESIAN_POINT('Ctrl Pts',(5.28717136811017,7.0076963147076,4.43657742893708));
#15000=CARTESIAN_POINT('Ctrl Pts',(5.06016846049025,6.98154572659498,4.20960102607602));
#15001=CARTESIAN_POINT('Ctrl Pts',(5.02365602163957,6.95531367050233,3.8895921954164));
#15002=CARTESIAN_POINT('Ctrl Pts',(5.19551794912881,6.92901180249481,3.61604266611656));
#15003=CARTESIAN_POINT('Ctrl Pts',(5.50106527788403,6.90264790572184,3.50895870577898));
#15004=CARTESIAN_POINT('Ctrl Pts',(5.79577161674239,6.87721212889977,3.61217861137834));
#15005=CARTESIAN_POINT('Ctrl Pts',(5.96305449537282,6.85271938331077,3.85785645038935));
#15006=CARTESIAN_POINT('Ctrl Pts',(5.96336129173779,6.82918177238479,4.14336056358693));
#15007=CARTESIAN_POINT('Ctrl Pts',(5.81582158193089,6.8075910527215,4.35981776235806));
#15008=CARTESIAN_POINT('Ctrl Pts',(5.60511420817303,6.78795692457779,4.46092931066051));
#15009=CARTESIAN_POINT('Ctrl Pts',(5.43000786563227,6.7732300740845,4.4609734353019));
#15010=CARTESIAN_POINT('Ctrl Pts',(5.30020839954856,6.76144926677095,4.41542525093647));
#15011=CARTESIAN_POINT('Ctrl Pts',(5.18374235150296,6.74966952273624,4.34235663912504));
#15012=CARTESIAN_POINT('Ctrl Pts',(5.07447092113825,6.73494816191923,4.20547111387009));
#15013=CARTESIAN_POINT('Ctrl Pts',(5.02784718599889,6.71729065774043,4.00065747110974));
#15014=CARTESIAN_POINT('Ctrl Pts',(5.07447386054353,6.69964459568449,3.79601025923107));
#15015=CARTESIAN_POINT('Ctrl Pts',(5.20529905681373,6.68201315439094,3.63204273671346));
#15016=CARTESIAN_POINT('Ctrl Pts',(5.39408590362551,6.66439961395901,3.54116301717729));
#15017=CARTESIAN_POINT('Ctrl Pts',(5.60333609396693,6.64680714416216,3.54119434056683));
#15018=CARTESIAN_POINT('Ctrl Pts',(5.7916924204204,6.62923879520195,3.63192246515604));
#15019=CARTESIAN_POINT('Ctrl Pts',(5.92158289603545,6.61169790649974,3.79506746854736));
#15020=CARTESIAN_POINT('Ctrl Pts',(5.97348422705736,6.59224132115423,4.0208010865485));
#15021=CARTESIAN_POINT('Ctrl Pts',(5.89702584711254,6.57088802899332,4.2682427919361));
#15022=CARTESIAN_POINT('Ctrl Pts',(5.69487546676521,6.54959462586925,4.42916632782277));
#15023=CARTESIAN_POINT('Ctrl Pts',(5.51317481886798,6.53415151193397,4.45613715780873));
#15024=CARTESIAN_POINT('Ctrl Pts',(5.35801698637868,6.52066195925173,4.43279204584114));
#15025=CARTESIAN_POINT('Ctrl Pts',(5.21374009576453,6.50719519620621,4.36329408523511));
#15026=CARTESIAN_POINT('Ctrl Pts',(5.08567798395226,6.48992954163975,4.20264939874256));
#15027=CARTESIAN_POINT('Ctrl Pts',(5.04041661933432,6.47271281314042,4.00302390822556));
#15028=CARTESIAN_POINT('Ctrl Pts',(5.09312070125709,6.45268959111598,3.770743151734));
#15029=CARTESIAN_POINT('Ctrl Pts',(5.29058645351125,6.42989526702207,3.57256208940533));
#15030=CARTESIAN_POINT('Ctrl Pts',(5.56736489827577,6.40722162609742,3.54199581368896));
#15031=CARTESIAN_POINT('Ctrl Pts',(5.76353539464181,6.38888263494561,3.63733190145256));
#15032=CARTESIAN_POINT('Ctrl Pts',(5.89598723312259,6.37201371483763,3.78518032709043));
#15033=CARTESIAN_POINT('Ctrl Pts',(5.94748358103074,6.35660808187041,3.96374439081115));
#15034=CARTESIAN_POINT('Ctrl Pts',(5.91685865376627,6.34126760667545,4.14161364905986));
#15035=CARTESIAN_POINT('Ctrl Pts',(5.82224248057764,6.32458502365897,4.31366053046754));
#15036=CARTESIAN_POINT('Ctrl Pts',(5.60660953292401,6.30382997132046,4.44913008611416));
#15037=CARTESIAN_POINT('Ctrl Pts',(5.30470259158896,6.27909158348978,4.41475311910331));
#15038=CARTESIAN_POINT('Ctrl Pts',(5.09170051369519,6.25452341621551,4.20123511708807));
#15039=CARTESIAN_POINT('Ctrl Pts',(5.05856247602295,6.23013365457353,3.90374222299026));
#15040=CARTESIAN_POINT('Ctrl Pts',(5.21710547478983,6.20591600947063,3.65215819590566));
#15041=CARTESIAN_POINT('Ctrl Pts',(5.4955522329887,6.18189025349015,3.55516775542111));
#15042=CARTESIAN_POINT('Ctrl Pts',(5.72567785231775,6.16201826770261,3.63598206917989));
#15043=CARTESIAN_POINT('Ctrl Pts',(5.82854913820436,6.14885155715524,3.75185257807874));
#15044=CARTESIAN_POINT('Ctrl Pts',(5.88768132090037,6.13834655444601,3.85862649586901));
#15045=CARTESIAN_POINT('Ctrl Pts',(5.91865398757851,6.12656716972265,3.99513809825376));
#15046=CARTESIAN_POINT('Ctrl Pts',(5.87056737474013,6.10834280183518,4.20678461191633));
#15047=CARTESIAN_POINT('Ctrl Pts',(5.72480600833643,6.09153123535025,4.35234929299144));
#15048=CARTESIAN_POINT('Ctrl Pts',(5.55008041460532,6.07610979937891,4.40202024202591));
#15049=CARTESIAN_POINT('Ctrl Pts',(5.39986618875751,6.06331159280831,4.3937717269471));
#15050=CARTESIAN_POINT('Ctrl Pts',(5.24977367075476,6.04930117532489,4.32130130885873));
#15051=CARTESIAN_POINT('Ctrl Pts',(5.1370759222932,6.03410042382611,4.17994965722586));
#15052=CARTESIAN_POINT('Ctrl Pts',(5.09722624552166,6.0189859086027,4.00464345758488));
#15053=CARTESIAN_POINT('Ctrl Pts',(5.13708274489156,6.00395199588207,3.83031021460055));
#15054=CARTESIAN_POINT('Ctrl Pts',(5.24808791700962,5.98900127852958,3.6914414666054));
#15055=CARTESIAN_POINT('Ctrl Pts',(5.40745664968594,5.97413206983575,3.61467943867966));
#15056=CARTESIAN_POINT('Ctrl Pts',(5.55399870251856,5.96180976298947,3.61486056493999));
#15057=CARTESIAN_POINT('Ctrl Pts',(5.64862248135238,5.95321954864974,3.6480666103073));
#15058=CARTESIAN_POINT('Ctrl Pts',(5.69842524536096,5.94832094967742,3.67559303366571));
#15059=CARTESIAN_POINT('Ctrl Pts',(5.76798070022639,5.94098275227965,3.72490537830438));
#15060=CARTESIAN_POINT('Ctrl Pts',(5.84923025676308,5.93001063189764,3.82698024714553));
#15061=CARTESIAN_POINT('Ctrl Pts',(5.88773532824436,5.91545880053051,3.99575027454172));
#15062=CARTESIAN_POINT('Ctrl Pts',(5.84925547744142,5.9009828238771,4.1635444551542));
#15063=CARTESIAN_POINT('Ctrl Pts',(5.7513255464219,5.88778222195693,4.28630739949125));
#15064=CARTESIAN_POINT('Ctrl Pts',(5.6282755026934,5.87583551525214,4.35409079257078));
#15065=CARTESIAN_POINT('Ctrl Pts',(5.46253669380234,5.86155308506761,4.38260610594922));
#15066=CARTESIAN_POINT('Ctrl Pts',(5.25709446927773,5.84379840048457,4.31056950119396));
#15067=CARTESIAN_POINT('Ctrl Pts',(5.1188863731938,5.8226444314236,4.09047085545772));
#15068=CARTESIAN_POINT('Ctrl Pts',(5.14821797566417,5.80163306758262,3.83419489648604));
#15069=CARTESIAN_POINT('Ctrl Pts',(5.32948302926564,5.78076121516305,3.65319222396216));
#15070=CARTESIAN_POINT('Ctrl Pts',(5.58272277651973,5.76001882939718,3.62490963002238));
#15071=CARTESIAN_POINT('Ctrl Pts',(5.76094172440336,5.74283538634389,3.73734906526789));
#15072=CARTESIAN_POINT('Ctrl Pts',(5.83858054429191,5.72914477225272,3.8785842544305));
#15073=CARTESIAN_POINT('Ctrl Pts',(5.8520911023979,5.72232128177237,3.95760364160119));
#15074=CARTESIAN_POINT('Ctrl Pts',(5.85209646263188,5.71890639514741,3.99733391297083));
#15075=CARTESIAN_POINT('Ctrl Pts',(5.9149593871984,7.09981632447119,4.00428381887363));
#15076=CARTESIAN_POINT('Ctrl Pts',(5.91495308543952,7.0958016186183,4.05099264708924));
#15077=CARTESIAN_POINT('Ctrl Pts',(5.89904039139162,7.08776451910168,4.14406609975579));
#15078=CARTESIAN_POINT('Ctrl Pts',(5.80762376136514,7.07163070606742,4.31058337466593));
#15079=CARTESIAN_POINT('Ctrl Pts',(5.59721423545493,7.05136306306487,4.44307682955313));
#15080=CARTESIAN_POINT('Ctrl Pts',(5.29839493635342,7.02688072250891,4.40985935994832));
#15081=CARTESIAN_POINT('Ctrl Pts',(5.08441495345513,7.00224296763148,4.19612662281291));
#15082=CARTESIAN_POINT('Ctrl Pts',(5.04974875241047,6.97745444355743,3.89375224127796));
#15083=CARTESIAN_POINT('Ctrl Pts',(5.21250981495705,6.95252140927353,3.63434621044489));
#15084=CARTESIAN_POINT('Ctrl Pts',(5.50304341273993,6.9274480281682,3.5323300193668));
#15085=CARTESIAN_POINT('Ctrl Pts',(5.78434555072646,6.90317511570346,3.6306649383391));
#15086=CARTESIAN_POINT('Ctrl Pts',(5.94463823132403,6.87972443166664,3.86582463725867));
#15087=CARTESIAN_POINT('Ctrl Pts',(5.94506874025421,6.85711505479382,4.14007773066394));
#15088=CARTESIAN_POINT('Ctrl Pts',(5.80298180027145,6.83630820453566,4.34876669420255));
#15089=CARTESIAN_POINT('Ctrl Pts',(5.5993330098206,6.81733128287079,4.44656967130991));
#15090=CARTESIAN_POINT('Ctrl Pts',(5.42963725623126,6.80306132062808,4.44666183830942));
#15091=CARTESIAN_POINT('Ctrl Pts',(5.30359323362781,6.79162260587336,4.40244344229727));
#15092=CARTESIAN_POINT('Ctrl Pts',(5.19034833118513,6.78016936879213,4.33140732330614));
#15093=CARTESIAN_POINT('Ctrl Pts',(5.08385604486381,6.76583190694975,4.19809246217554));
#15094=CARTESIAN_POINT('Ctrl Pts',(5.03825146773315,6.74858505106259,3.99803805883399));
#15095=CARTESIAN_POINT('Ctrl Pts',(5.08385657844574,6.73130389443769,3.79758257367279));
#15096=CARTESIAN_POINT('Ctrl Pts',(5.21228621879808,6.71399268838207,3.63650910211638));
#15097=CARTESIAN_POINT('Ctrl Pts',(5.39817377695134,6.69665086519213,3.54694964375529));
#15098=CARTESIAN_POINT('Ctrl Pts',(5.60480938276286,6.67928251587732,3.54691321479687));
#15099=CARTESIAN_POINT('Ctrl Pts',(5.79136032917417,6.66189043106636,3.63669165399195));
#15100=CARTESIAN_POINT('Ctrl Pts',(5.92039378666778,6.64447639659799,3.798656873621));
#15101=CARTESIAN_POINT('Ctrl Pts',(5.97215579848303,6.62510974481235,4.02340656085786));
#15102=CARTESIAN_POINT('Ctrl Pts',(5.89590223862252,6.60377676600798,4.27066947166225));
#15103=CARTESIAN_POINT('Ctrl Pts',(5.69328362721486,6.58243024014988,4.43216184340459));
#15104=CARTESIAN_POINT('Ctrl Pts',(5.51047755263859,6.56689647414804,4.45935690682349));
#15105=CARTESIAN_POINT('Ctrl Pts',(5.35407501259111,6.5533004896361,4.43583123820807));
#15106=CARTESIAN_POINT('Ctrl Pts',(5.20835461031678,6.53970490291349,4.36569371401464));
#15107=CARTESIAN_POINT('Ctrl Pts',(5.07860298299557,6.52221993385381,4.20304133979497));
#15108=CARTESIAN_POINT('Ctrl Pts',(5.03257499448107,6.50474274920277,4.00032758858315));
#15109=CARTESIAN_POINT('Ctrl Pts',(5.08616781619013,6.48435453861134,3.76376359272689));
#15110=CARTESIAN_POINT('Ctrl Pts',(5.28778842673841,6.46107782796493,3.56112334924671));
#15111=CARTESIAN_POINT('Ctrl Pts',(5.57177694710294,6.43781826428389,3.52956237290512));
#15112=CARTESIAN_POINT('Ctrl Pts',(5.77378591102479,6.4189467241674,3.62766025014304));
#15113=CARTESIAN_POINT('Ctrl Pts',(5.91050945448788,6.40153607632419,3.78023093558462));
#15114=CARTESIAN_POINT('Ctrl Pts',(5.96387927126282,6.38560528324312,3.96495886197815));
#15115=CARTESIAN_POINT('Ctrl Pts',(5.93213495257581,6.36969190270551,4.14951323780822));
#15116=CARTESIAN_POINT('Ctrl Pts',(5.83381323704975,6.35235284740185,4.32837272892742));
#15117=CARTESIAN_POINT('Ctrl Pts',(5.60911648444059,6.33072654274578,4.46973537115468));
#15118=CARTESIAN_POINT('Ctrl Pts',(5.2931718071227,6.30484798080865,4.43396198639303));
#15119=CARTESIAN_POINT('Ctrl Pts',(5.06932425874092,6.27905716144787,4.20984555330695));
#15120=CARTESIAN_POINT('Ctrl Pts',(5.03421828644466,6.25335480389872,3.89629859927553));
#15121=CARTESIAN_POINT('Ctrl Pts',(5.20171418169518,6.22777084145329,3.63015017227696));
#15122=CARTESIAN_POINT('Ctrl Pts',(5.49713289769245,6.2022789177778,3.52707275798132));
#15123=CARTESIAN_POINT('Ctrl Pts',(5.74210439555382,6.18114457050484,3.61295915765088));
#15124=CARTESIAN_POINT('Ctrl Pts',(5.8518682951323,6.16710129700844,3.7365649924753));
#15125=CARTESIAN_POINT('Ctrl Pts',(5.91501706249361,6.15588489652694,3.85058437438587));
#15126=CARTESIAN_POINT('Ctrl Pts',(5.94815875179138,6.1432946488714,3.99652625741968));
#15127=CARTESIAN_POINT('Ctrl Pts',(5.89670996174374,6.12377785850373,4.22323046031872));
#15128=CARTESIAN_POINT('Ctrl Pts',(5.74032627079256,6.10574426054262,4.37953203223293));
#15129=CARTESIAN_POINT('Ctrl Pts',(5.55243898812676,6.08916696227491,4.4329671523606));
#15130=CARTESIAN_POINT('Ctrl Pts',(5.39071604519891,6.07539302167999,4.42410346032364));
#15131=CARTESIAN_POINT('Ctrl Pts',(5.22890883093779,6.0602953077351,4.34599909074473));
#15132=CARTESIAN_POINT('Ctrl Pts',(5.10722454589011,6.04389396153373,4.19343552007192));
#15133=CARTESIAN_POINT('Ctrl Pts',(5.06413039868302,6.02755830971277,4.00393860928497));
#15134=CARTESIAN_POINT('Ctrl Pts',(5.10722831777621,6.01129684192045,3.81527822605878));
#15135=CARTESIAN_POINT('Ctrl Pts',(5.22747548470254,5.995106342901,3.66482621676792));
#15136=CARTESIAN_POINT('Ctrl Pts',(5.40028163714302,5.97898878411569,3.58156898328027));
#15137=CARTESIAN_POINT('Ctrl Pts',(5.55933969240477,5.96561723512518,3.58175740628002));
#15138=CARTESIAN_POINT('Ctrl Pts',(5.66210550300135,5.9562890894632,3.61781790440772));
#15139=CARTESIAN_POINT('Ctrl Pts',(5.71620838528512,5.95096787527999,3.64772140297022));
#15140=CARTESIAN_POINT('Ctrl Pts',(5.79178201838636,5.94299563414587,3.70129807305379));
#15141=CARTESIAN_POINT('Ctrl Pts',(5.88009213765861,5.93107477634743,3.81223105667651));
#15142=CARTESIAN_POINT('Ctrl Pts',(5.92197627191235,5.91525578799805,3.99574650770481));
#15143=CARTESIAN_POINT('Ctrl Pts',(5.88011310439625,5.89951367020608,4.17827551464281));
#15144=CARTESIAN_POINT('Ctrl Pts',(5.77355284379942,5.88515292216243,4.31185923524939));
#15145=CARTESIAN_POINT('Ctrl Pts',(5.63963221810424,5.87215333951234,4.38562554412733));
#15146=CARTESIAN_POINT('Ctrl Pts',(5.45924850580616,5.85661192507217,4.41665712792164));
#15147=CARTESIAN_POINT('Ctrl Pts',(5.23567580323262,5.83729458949201,4.33824620829054));
#15148=CARTESIAN_POINT('Ctrl Pts',(5.08534542689851,5.81428812401155,4.09879386786708));
#15149=CARTESIAN_POINT('Ctrl Pts',(5.11727898328737,5.79145701238181,3.8202071105913));
#15150=CARTESIAN_POINT('Ctrl Pts',(5.31417199281544,5.76879711912542,3.62367687736167));
#15151=CARTESIAN_POINT('Ctrl Pts',(5.58884524217245,5.74630623137894,3.59308087302305));
#15152=CARTESIAN_POINT('Ctrl Pts',(5.78177453472185,5.72770685157949,3.71490177588423));
#15153=CARTESIAN_POINT('Ctrl Pts',(5.86570779175526,5.71290424187196,3.86762747609063));
#15154=CARTESIAN_POINT('Ctrl Pts',(5.88029185858757,5.70553413368606,3.95299047765566));
#15155=CARTESIAN_POINT('Ctrl Pts',(5.88029764289545,5.7018490789545,3.99586400189707));
#15156=CARTESIAN_POINT('Ctrl Pts',(5.89999942231746,7.09981632447119,4.00428180053801));
#15157=CARTESIAN_POINT('Ctrl Pts',(5.89999334367971,7.09594376396835,4.04933684813297));
#15158=CARTESIAN_POINT('Ctrl Pts',(5.88465017335476,7.08819405075721,4.13908165517953));
#15159=CARTESIAN_POINT('Ctrl Pts',(5.7964860030169,7.07263331806119,4.29968204261715));
#15160=CARTESIAN_POINT('Ctrl Pts',(5.59351456200701,7.05308119240215,4.4275031391656));
#15161=CARTESIAN_POINT('Ctrl Pts',(5.30510775645105,7.02945158726801,4.39546636939848));
#15162=CARTESIAN_POINT('Ctrl Pts',(5.09844717527872,7.00565845259414,4.18908156433879));
#15163=CARTESIAN_POINT('Ctrl Pts',(5.06491507736497,6.98170283632427,3.89688445847127));
#15164=CARTESIAN_POINT('Ctrl Pts',(5.22229231109316,6.957587725778,3.64598811283775));
#15165=CARTESIAN_POINT('Ctrl Pts',(5.50350105188817,6.93331581944121,3.54720017800962));
#15166=CARTESIAN_POINT('Ctrl Pts',(5.77606730494162,6.90979543600253,3.64243302852389));
#15167=CARTESIAN_POINT('Ctrl Pts',(5.93155863446605,6.88704927881041,3.87048202703801));
#15168=CARTESIAN_POINT('Ctrl Pts',(5.93201459027321,6.86509833940111,4.13672884061229));
#15169=CARTESIAN_POINT('Ctrl Pts',(5.79395734371705,6.84487476341531,4.33956419787309));
#15170=CARTESIAN_POINT('Ctrl Pts',(5.59585169142646,6.82641140225049,4.43472796239094));
#15171=CARTESIAN_POINT('Ctrl Pts',(5.43062330290708,6.81251496798271,4.43483227755276));
#15172=CARTESIAN_POINT('Ctrl Pts',(5.30781628774365,6.8013693608627,4.39175312056372));
#15173=CARTESIAN_POINT('Ctrl Pts',(5.19743069189207,6.79020509173472,4.32251414855249));
#15174=CARTESIAN_POINT('Ctrl Pts',(5.09353798605695,6.77621535562195,4.1924772803632));
#15175=CARTESIAN_POINT('Ctrl Pts',(5.04898925851302,6.75937456735607,3.99715324700454));
#15176=CARTESIAN_POINT('Ctrl Pts',(5.0935413464267,6.74248271039737,3.80123524176677));
#15177=CARTESIAN_POINT('Ctrl Pts',(5.21917592334569,6.72554188446977,3.64363320271165));
#15178=CARTESIAN_POINT('Ctrl Pts',(5.40122000385758,6.70855426693318,3.55590244763416));
#15179=CARTESIAN_POINT('Ctrl Pts',(5.60380955719718,6.6915221019177,3.55584448787041));
#15180=CARTESIAN_POINT('Ctrl Pts',(5.78691645390742,6.67444770371231,3.64394104146688));
#15181=CARTESIAN_POINT('Ctrl Pts',(5.91372041331327,6.65733344366189,3.80307026683985));
#15182=CARTESIAN_POINT('Ctrl Pts',(5.96466327221314,6.63827601600008,4.02414934139344));
#15183=CARTESIAN_POINT('Ctrl Pts',(5.88961383686182,6.61726302422527,4.26770951451258));
#15184=CARTESIAN_POINT('Ctrl Pts',(5.68975602864846,6.59619863118807,4.42707389952551));
#15185=CARTESIAN_POINT('Ctrl Pts',(5.50916223586277,6.58084997697241,4.45396467698472));
#15186=CARTESIAN_POINT('Ctrl Pts',(5.35453310810722,6.56740673736238,4.43070717074375));
#15187=CARTESIAN_POINT('Ctrl Pts',(5.21033393748589,6.55395079494006,4.36132595428699));
#15188=CARTESIAN_POINT('Ctrl Pts',(5.08177516019845,6.53662851034176,4.20021226638331));
#15189=CARTESIAN_POINT('Ctrl Pts',(5.03609211123456,6.51928717867399,3.99913913108666));
#15190=CARTESIAN_POINT('Ctrl Pts',(5.08928582945947,6.49903664031616,3.76419897777231));
#15191=CARTESIAN_POINT('Ctrl Pts',(5.28978283301087,6.47587070029814,3.56256415950519));
#15192=CARTESIAN_POINT('Ctrl Pts',(5.57279015344961,6.4526862562021,3.53101713469425));
#15193=CARTESIAN_POINT('Ctrl Pts',(5.7744501239661,6.4338421384389,3.62890875798563));
#15194=CARTESIAN_POINT('Ctrl Pts',(5.91107614262552,6.41644569471267,3.78134048060785));
#15195=CARTESIAN_POINT('Ctrl Pts',(5.96451577569518,6.40049895608791,3.96616344909838));
#15196=CARTESIAN_POINT('Ctrl Pts',(5.9327299609379,6.3845554854669,4.15104965949736));
#15197=CARTESIAN_POINT('Ctrl Pts',(5.83415684595966,6.36716688464879,4.33040203531341));
#15198=CARTESIAN_POINT('Ctrl Pts',(5.60855787080152,6.3454421500065,4.47243154476512));
#15199=CARTESIAN_POINT('Ctrl Pts',(5.29067075546292,6.31939963984916,4.43654609473001));
#15200=CARTESIAN_POINT('Ctrl Pts',(5.06495666340114,6.29339375333233,4.21070709279472));
#15201=CARTESIAN_POINT('Ctrl Pts',(5.02940089438198,6.26743382198568,3.89407398616837));
#15202=CARTESIAN_POINT('Ctrl Pts',(5.19880065125732,6.24152902171826,3.62471661866899));
#15203=CARTESIAN_POINT('Ctrl Pts',(5.49820781434257,6.21568834443117,3.52014376389726));
#15204=CARTESIAN_POINT('Ctrl Pts',(5.74701061020189,6.19421520170402,3.60728770872527));
#15205=CARTESIAN_POINT('Ctrl Pts',(5.85863359577984,6.17993370216935,3.73296424281348));
#15206=CARTESIAN_POINT('Ctrl Pts',(5.92288006435656,6.16852118154694,3.84896516413552));
#15207=CARTESIAN_POINT('Ctrl Pts',(5.95664235896203,6.15570021350747,3.99755228818456));
#15208=CARTESIAN_POINT('Ctrl Pts',(5.90422907170185,6.13580438066566,4.22863954557107));
#15209=CARTESIAN_POINT('Ctrl Pts',(5.74463079333177,6.1173884553624,4.38823789360272));
#15210=CARTESIAN_POINT('Ctrl Pts',(5.55259803695828,6.10044178794059,4.44287010078724));
#15211=CARTESIAN_POINT('Ctrl Pts',(5.38717753744307,6.08634982964905,4.43381260797737));
#15212=CARTESIAN_POINT('Ctrl Pts',(5.22149962135128,6.07088880373497,4.35387124517548));
#15213=CARTESIAN_POINT('Ctrl Pts',(5.09676922730111,6.0540743240685,4.197519449458));
#15214=CARTESIAN_POINT('Ctrl Pts',(5.0525318165955,6.03731392845979,4.00312051246728));
#15215=CARTESIAN_POINT('Ctrl Pts',(5.09677460214568,6.02060952469266,3.80936725739853));
#15216=CARTESIAN_POINT('Ctrl Pts',(5.22036100773764,6.00396293698029,3.65469518694587));
#15217=CARTESIAN_POINT('Ctrl Pts',(5.39815221757406,5.98737590584214,3.56901265908242));
#15218=CARTESIAN_POINT('Ctrl Pts',(5.56194673621828,5.9736043825902,3.56918712785721));
#15219=CARTESIAN_POINT('Ctrl Pts',(5.6678409475086,5.96399177625527,3.60634259138081));
#15220=CARTESIAN_POINT('Ctrl Pts',(5.72360710674561,5.9585067948969,3.63716464071472));
#15221=CARTESIAN_POINT('Ctrl Pts',(5.80152037634414,5.9502873075744,3.69239994875946));
#15222=CARTESIAN_POINT('Ctrl Pts',(5.89262775771971,5.93798818799799,3.80682412790902));
#15223=CARTESIAN_POINT('Ctrl Pts',(5.93588165070209,5.9216549676263,3.9962737943898));
#15224=CARTESIAN_POINT('Ctrl Pts',(5.89265315890838,5.90538862230925,4.18485446150754));
#15225=CARTESIAN_POINT('Ctrl Pts',(5.78249899819111,5.89054018760752,4.32296861862104));
#15226=CARTESIAN_POINT('Ctrl Pts',(5.64397324912796,5.87709200642215,4.39928196165792));
#15227=CARTESIAN_POINT('Ctrl Pts',(5.45729571883929,5.86100659113963,4.43140768516966));
#15228=CARTESIAN_POINT('Ctrl Pts',(5.22574876053333,5.84099901355926,4.35024097908663));
#15229=CARTESIAN_POINT('Ctrl Pts',(5.0699063365284,5.81715142001874,4.10208650989737));
#15230=CARTESIAN_POINT('Ctrl Pts',(5.10298913581097,5.79346725679344,3.81314318112568));
#15231=CARTESIAN_POINT('Ctrl Pts',(5.30729513304354,5.76994860790156,3.60917536341897));
#15232=CARTESIAN_POINT('Ctrl Pts',(5.59246492988907,5.74659517888843,3.57738640664907));
#15233=CARTESIAN_POINT('Ctrl Pts',(5.79284572265032,5.72727468967069,3.7038989587173));
#15234=CARTESIAN_POINT('Ctrl Pts',(5.8800308145667,5.71189869700794,3.86253471396896));
#15235=CARTESIAN_POINT('Ctrl Pts',(5.8951821641861,5.70424160396714,3.95121652410008));
#15236=CARTESIAN_POINT('Ctrl Pts',(5.89518817092524,5.70041484319491,3.99573871784903));
#15237=CARTESIAN_POINT('',(5.89999942231746,7.09981632447119,4.00428180053802));
#15238=CARTESIAN_POINT('Origin',(5.9,7.05,4.));
#15239=CARTESIAN_POINT('',(5.89518817092524,5.70041484319491,3.99573871784901));
#15240=CARTESIAN_POINT('Ctrl Pts',(5.89999942231746,7.09981632447119,4.00428180053801));
#15241=CARTESIAN_POINT('Ctrl Pts',(5.89999334367971,7.09594376396835,4.04933684813297));
#15242=CARTESIAN_POINT('Ctrl Pts',(5.88465017335476,7.08819405075721,4.13908165517953));
#15243=CARTESIAN_POINT('Ctrl Pts',(5.7964860030169,7.07263331806119,4.29968204261715));
#15244=CARTESIAN_POINT('Ctrl Pts',(5.59351456200701,7.05308119240215,4.4275031391656));
#15245=CARTESIAN_POINT('Ctrl Pts',(5.30510775645105,7.02945158726801,4.39546636939848));
#15246=CARTESIAN_POINT('Ctrl Pts',(5.09844717527872,7.00565845259414,4.18908156433879));
#15247=CARTESIAN_POINT('Ctrl Pts',(5.06491507736497,6.98170283632427,3.89688445847127));
#15248=CARTESIAN_POINT('Ctrl Pts',(5.22229231109316,6.957587725778,3.64598811283775));
#15249=CARTESIAN_POINT('Ctrl Pts',(5.50350105188817,6.93331581944121,3.54720017800962));
#15250=CARTESIAN_POINT('Ctrl Pts',(5.77606730494162,6.90979543600253,3.64243302852389));
#15251=CARTESIAN_POINT('Ctrl Pts',(5.93155863446605,6.88704927881041,3.87048202703801));
#15252=CARTESIAN_POINT('Ctrl Pts',(5.93201459027321,6.86509833940111,4.13672884061229));
#15253=CARTESIAN_POINT('Ctrl Pts',(5.79395734371705,6.84487476341531,4.33956419787309));
#15254=CARTESIAN_POINT('Ctrl Pts',(5.59585169142646,6.82641140225049,4.43472796239094));
#15255=CARTESIAN_POINT('Ctrl Pts',(5.43062330290708,6.81251496798271,4.43483227755276));
#15256=CARTESIAN_POINT('Ctrl Pts',(5.30781628774365,6.8013693608627,4.39175312056372));
#15257=CARTESIAN_POINT('Ctrl Pts',(5.19743069189207,6.79020509173472,4.32251414855249));
#15258=CARTESIAN_POINT('Ctrl Pts',(5.09353798605695,6.77621535562195,4.1924772803632));
#15259=CARTESIAN_POINT('Ctrl Pts',(5.04898925851302,6.75937456735607,3.99715324700454));
#15260=CARTESIAN_POINT('Ctrl Pts',(5.0935413464267,6.74248271039737,3.80123524176677));
#15261=CARTESIAN_POINT('Ctrl Pts',(5.21917592334569,6.72554188446977,3.64363320271165));
#15262=CARTESIAN_POINT('Ctrl Pts',(5.40122000385758,6.70855426693318,3.55590244763416));
#15263=CARTESIAN_POINT('Ctrl Pts',(5.60380955719718,6.6915221019177,3.55584448787041));
#15264=CARTESIAN_POINT('Ctrl Pts',(5.78691645390742,6.67444770371231,3.64394104146688));
#15265=CARTESIAN_POINT('Ctrl Pts',(5.91372041331327,6.65733344366189,3.80307026683985));
#15266=CARTESIAN_POINT('Ctrl Pts',(5.96466327221314,6.63827601600008,4.02414934139344));
#15267=CARTESIAN_POINT('Ctrl Pts',(5.88961383686182,6.61726302422527,4.26770951451258));
#15268=CARTESIAN_POINT('Ctrl Pts',(5.68975602864846,6.59619863118807,4.42707389952551));
#15269=CARTESIAN_POINT('Ctrl Pts',(5.50916223586277,6.58084997697241,4.45396467698472));
#15270=CARTESIAN_POINT('Ctrl Pts',(5.35453310810722,6.56740673736238,4.43070717074375));
#15271=CARTESIAN_POINT('Ctrl Pts',(5.21033393748589,6.55395079494006,4.36132595428699));
#15272=CARTESIAN_POINT('Ctrl Pts',(5.08177516019845,6.53662851034176,4.20021226638331));
#15273=CARTESIAN_POINT('Ctrl Pts',(5.03609211123456,6.51928717867399,3.99913913108666));
#15274=CARTESIAN_POINT('Ctrl Pts',(5.08928582945947,6.49903664031616,3.76419897777231));
#15275=CARTESIAN_POINT('Ctrl Pts',(5.28978283301087,6.47587070029814,3.56256415950519));
#15276=CARTESIAN_POINT('Ctrl Pts',(5.57279015344961,6.4526862562021,3.53101713469425));
#15277=CARTESIAN_POINT('Ctrl Pts',(5.7744501239661,6.4338421384389,3.62890875798563));
#15278=CARTESIAN_POINT('Ctrl Pts',(5.91107614262552,6.41644569471267,3.78134048060785));
#15279=CARTESIAN_POINT('Ctrl Pts',(5.96451577569518,6.40049895608791,3.96616344909838));
#15280=CARTESIAN_POINT('Ctrl Pts',(5.9327299609379,6.3845554854669,4.15104965949736));
#15281=CARTESIAN_POINT('Ctrl Pts',(5.83415684595966,6.36716688464879,4.33040203531341));
#15282=CARTESIAN_POINT('Ctrl Pts',(5.60855787080152,6.3454421500065,4.47243154476512));
#15283=CARTESIAN_POINT('Ctrl Pts',(5.29067075546292,6.31939963984916,4.43654609473001));
#15284=CARTESIAN_POINT('Ctrl Pts',(5.06495666340114,6.29339375333233,4.21070709279472));
#15285=CARTESIAN_POINT('Ctrl Pts',(5.02940089438198,6.26743382198568,3.89407398616837));
#15286=CARTESIAN_POINT('Ctrl Pts',(5.19880065125732,6.24152902171826,3.62471661866899));
#15287=CARTESIAN_POINT('Ctrl Pts',(5.49820781434257,6.21568834443117,3.52014376389726));
#15288=CARTESIAN_POINT('Ctrl Pts',(5.74701061020189,6.19421520170402,3.60728770872527));
#15289=CARTESIAN_POINT('Ctrl Pts',(5.85863359577984,6.17993370216935,3.73296424281348));
#15290=CARTESIAN_POINT('Ctrl Pts',(5.92288006435656,6.16852118154694,3.84896516413552));
#15291=CARTESIAN_POINT('Ctrl Pts',(5.95664235896203,6.15570021350747,3.99755228818456));
#15292=CARTESIAN_POINT('Ctrl Pts',(5.90422907170185,6.13580438066566,4.22863954557107));
#15293=CARTESIAN_POINT('Ctrl Pts',(5.74463079333177,6.1173884553624,4.38823789360272));
#15294=CARTESIAN_POINT('Ctrl Pts',(5.55259803695828,6.10044178794059,4.44287010078724));
#15295=CARTESIAN_POINT('Ctrl Pts',(5.38717753744307,6.08634982964905,4.43381260797737));
#15296=CARTESIAN_POINT('Ctrl Pts',(5.22149962135128,6.07088880373497,4.35387124517548));
#15297=CARTESIAN_POINT('Ctrl Pts',(5.09676922730111,6.0540743240685,4.197519449458));
#15298=CARTESIAN_POINT('Ctrl Pts',(5.0525318165955,6.03731392845979,4.00312051246728));
#15299=CARTESIAN_POINT('Ctrl Pts',(5.09677460214568,6.02060952469266,3.80936725739853));
#15300=CARTESIAN_POINT('Ctrl Pts',(5.22036100773764,6.00396293698029,3.65469518694587));
#15301=CARTESIAN_POINT('Ctrl Pts',(5.39815221757406,5.98737590584214,3.56901265908242));
#15302=CARTESIAN_POINT('Ctrl Pts',(5.56194673621828,5.9736043825902,3.56918712785721));
#15303=CARTESIAN_POINT('Ctrl Pts',(5.6678409475086,5.96399177625527,3.60634259138081));
#15304=CARTESIAN_POINT('Ctrl Pts',(5.72360710674561,5.9585067948969,3.63716464071472));
#15305=CARTESIAN_POINT('Ctrl Pts',(5.80152037634414,5.9502873075744,3.69239994875946));
#15306=CARTESIAN_POINT('Ctrl Pts',(5.89262775771971,5.93798818799799,3.80682412790902));
#15307=CARTESIAN_POINT('Ctrl Pts',(5.93588165070209,5.9216549676263,3.9962737943898));
#15308=CARTESIAN_POINT('Ctrl Pts',(5.89265315890838,5.90538862230925,4.18485446150754));
#15309=CARTESIAN_POINT('Ctrl Pts',(5.78249899819111,5.89054018760752,4.32296861862104));
#15310=CARTESIAN_POINT('Ctrl Pts',(5.64397324912796,5.87709200642215,4.39928196165792));
#15311=CARTESIAN_POINT('Ctrl Pts',(5.45729571883929,5.86100659113963,4.43140768516966));
#15312=CARTESIAN_POINT('Ctrl Pts',(5.22574876053333,5.84099901355926,4.35024097908663));
#15313=CARTESIAN_POINT('Ctrl Pts',(5.0699063365284,5.81715142001874,4.10208650989737));
#15314=CARTESIAN_POINT('Ctrl Pts',(5.10298913581097,5.79346725679344,3.81314318112568));
#15315=CARTESIAN_POINT('Ctrl Pts',(5.30729513304354,5.76994860790156,3.60917536341897));
#15316=CARTESIAN_POINT('Ctrl Pts',(5.59246492988907,5.74659517888843,3.57738640664907));
#15317=CARTESIAN_POINT('Ctrl Pts',(5.79284572265032,5.72727468967069,3.7038989587173));
#15318=CARTESIAN_POINT('Ctrl Pts',(5.8800308145667,5.71189869700794,3.86253471396896));
#15319=CARTESIAN_POINT('Ctrl Pts',(5.8951821641861,5.70424160396714,3.95121652410008));
#15320=CARTESIAN_POINT('Ctrl Pts',(5.89518817092524,5.70041484319491,3.99573871784903));
#15321=CARTESIAN_POINT('Origin',(5.9,5.75,4.));
#15322=CARTESIAN_POINT('Origin',(5.9,5.75,4.));
#15323=CARTESIAN_POINT('Origin',(5.9,7.05,4.));
#16965=UNCERTAINTY_MEASURE_WITH_UNIT(LENGTH_MEASURE(0.001),#17047,
'DISTANCE_ACCURACY_VALUE',
'Maximum model space distance between geometric entities at asserted c
onnectivities');
#16993=UNCERTAINTY_MEASURE_WITH_UNIT(LENGTH_MEASURE(0.001),#17047,
'DISTANCE_ACCURACY_VALUE',
'Maximum model space distance between geometric entities at asserted c
onnectivities');
#17018=(
GEOMETRIC_REPRESENTATION_CONTEXT(3)
GLOBAL_UNCERTAINTY_ASSIGNED_CONTEXT((#16965))
GLOBAL_UNIT_ASSIGNED_CONTEXT((#17047,#17049,#17050))
REPRESENTATION_CONTEXT('','3D')
);
#17046=(
GEOMETRIC_REPRESENTATION_CONTEXT(3)
GLOBAL_UNCERTAINTY_ASSIGNED_CONTEXT((#16993))
GLOBAL_UNIT_ASSIGNED_CONTEXT((#17047,#17049,#17050))
REPRESENTATION_CONTEXT('','3D')
);
#17047=(
LENGTH_UNIT()
NAMED_UNIT(*)
SI_UNIT(.CENTI.,.METRE.)
);
#17049=(
NAMED_UNIT(*)
PLANE_ANGLE_UNIT()
SI_UNIT($,.RADIAN.)
);
#17050=(
NAMED_UNIT(*)
SI_UNIT($,.STERADIAN.)
SOLID_ANGLE_UNIT()
);
#17075=SHAPE_DEFINITION_REPRESENTATION(#17127,#17282);
#17127=PRODUCT_DEFINITION_SHAPE('',$,#17335);
#17282=SHAPE_REPRESENTATION('',(#9230),#17018);
#17310=PRODUCT_DEFINITION_CONTEXT('part definition',#17468,'design');
#17335=PRODUCT_DEFINITION('Preload spring (1)','Preload spring (1)',#17387,
#17310);
#17387=PRODUCT_DEFINITION_FORMATION('',$,#17494);
#17468=APPLICATION_CONTEXT(
'Core Data for Automotive Mechanical Design Process');
#17469=PRODUCT_CONTEXT('part definition',#17468,'mechanical');
#17494=PRODUCT('Preload spring (1)','Preload spring (1)','Preload spring (1)',
(#17469));
#17585=COLOUR_RGB('Grey',0.48,0.52,0.57);
#17586=FILL_AREA_STYLE_COLOUR('',#17585);
#17587=FILL_AREA_STYLE('',(#17586));
#17588=SURFACE_STYLE_FILL_AREA(#17587);
#17589=SURFACE_SIDE_STYLE('',(#17588));
#17590=SURFACE_STYLE_USAGE(.BOTH.,#17589);
#17591=PRESENTATION_STYLE_ASSIGNMENT((#17590));
ENDSEC;
END-ISO-10303-21;
